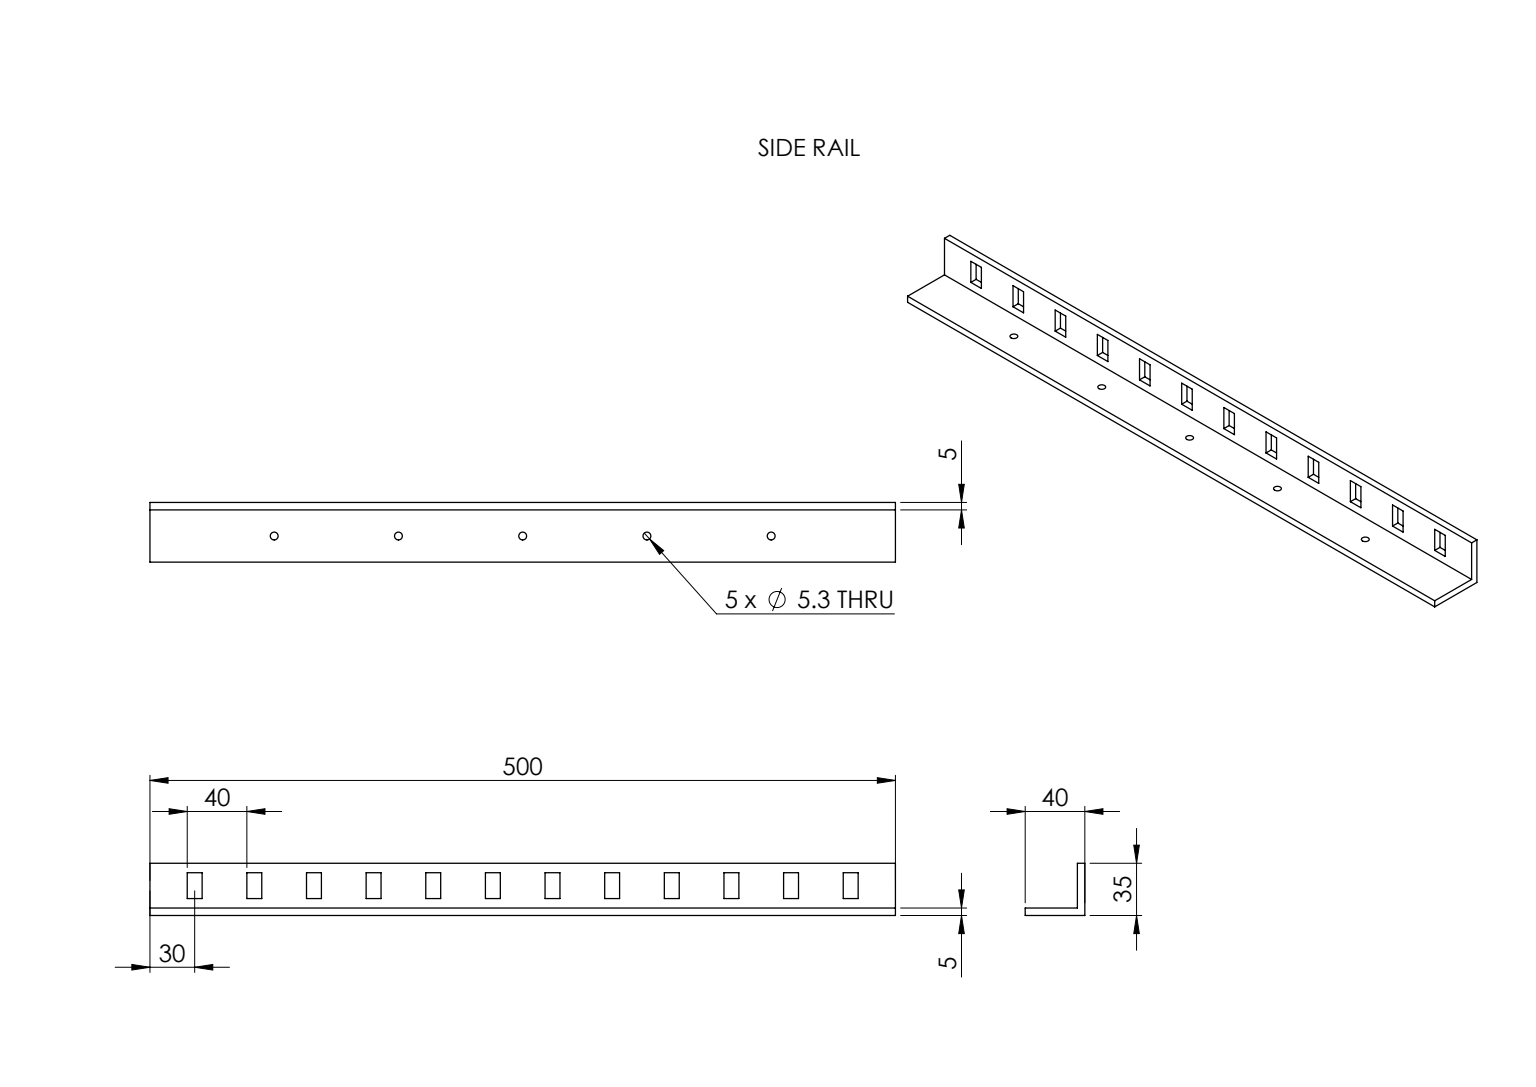
ISO-10303-21;
HEADER;
FILE_DESCRIPTION (('STEP AP214'),
    '1' );
FILE_NAME ('side rail.step',
    '2026-10-24T14:05:44',
    ( '' ),
    ( '' ),
    'SwSTEP 2.0',
    'SolidWorks 2026',
    '' );
FILE_SCHEMA (( 'AUTOMOTIVE_DESIGN' ));
ENDSEC;

DATA;
#4=CARTESIAN_POINT ( 'NONE',  ( 395.0000000000000000, -8.660254037844389075, 139.9990000000000236 ) ) ;
#6=EDGE_CURVE ( 'NONE', #1873, #4758, #4106, .T. ) ;
#9=CARTESIAN_POINT ( 'NONE',  ( 124.9999999999999858, 8.660254037844390851, 145.0000000000000284 ) ) ;
#13=EDGE_CURVE ( 'NONE', #2711, #3697, #5372, .T. ) ;
#15=DIRECTION ( 'NONE',  ( -0.000000000000000000, -0.000000000000000000, 1.000000000000000000 ) ) ;
#16=CARTESIAN_POINT ( 'NONE',  ( 395.0000000000000000, 8.660254037844390851, 140.0000000000000000 ) ) ;
#21=ORIENTED_EDGE ( 'NONE', *, *, #3815, .F. ) ;
#22=CARTESIAN_POINT ( 'NONE',  ( 445.0000000000000000, 8.660254037844390851, 145.0000000000000284 ) ) ;
#24=EDGE_CURVE ( 'NONE', #1078, #1538, #2930, .T. ) ;
#28=CARTESIAN_POINT ( 'NONE',  ( 285.0000000000000568, 8.660254037844390851, 139.9990000000000236 ) ) ;
#38=AXIS2_PLACEMENT_3D ( 'NONE', #3689, #2086, #340 ) ;
#39=DIRECTION ( 'NONE',  ( 0.000000000000000000, 0.000000000000000000, -1.000000000000000000 ) ) ;
#44=LINE ( 'NONE', #6748, #4124 ) ;
#49=CARTESIAN_POINT ( 'NONE',  ( 0.000000000000000000, -15.00000000000000000, 145.0000000000000284 ) ) ;
#50=CARTESIAN_POINT ( 'NONE',  ( 445.0000000000000000, 8.660254037844390851, 140.0000000000000000 ) ) ;
#54=EDGE_CURVE ( 'NONE', #6404, #2818, #2960, .T. ) ;
#58=VECTOR ( 'NONE', #6647, 1000.000000000000000 ) ;
#59=AXIS2_PLACEMENT_3D ( 'NONE', #3524, #1675, #1876 ) ;
#63=DIRECTION ( 'NONE',  ( 0.000000000000000000, -1.000000000000000000, 0.000000000000000000 ) ) ;
#67=EDGE_CURVE ( 'NONE', #3261, #4228, #2370, .T. ) ;
#74=LINE ( 'NONE', #2335, #4027 ) ;
#79=CARTESIAN_POINT ( 'NONE',  ( 303.3333333333333144, -20.00000000000000000, 162.5000000000000853 ) ) ;
#84=VERTEX_POINT ( 'NONE', #1298 ) ;
#90=CARTESIAN_POINT ( 'NONE',  ( 435.0000000000000568, 8.660254037844390851, 140.0000000000000000 ) ) ;
#92=ORIENTED_EDGE ( 'NONE', *, *, #7290, .F. ) ;
#95=ORIENTED_EDGE ( 'NONE', *, *, #13, .T. ) ;
#96=EDGE_CURVE ( 'NONE', #3309, #6744, #6473, .T. ) ;
#99=CARTESIAN_POINT ( 'NONE',  ( 155.0000000000000000, -8.660254037844389075, 139.9990000000000236 ) ) ;
#102=ORIENTED_EDGE ( 'NONE', *, *, #2735, .T. ) ;
#106=CARTESIAN_POINT ( 'NONE',  ( 155.0000000000000000, 8.660254037844390851, 140.0000000000000000 ) ) ;
#109=PLANE ( 'NONE',  #1833 ) ;
#110=DIRECTION ( 'NONE',  ( -0.000000000000000000, -0.000000000000000000, 1.000000000000000000 ) ) ;
#111=ORIENTED_EDGE ( 'NONE', *, *, #1690, .F. ) ;
#131=DIRECTION ( 'NONE',  ( 0.000000000000000000, -1.000000000000000000, 0.000000000000000000 ) ) ;
#133=VECTOR ( 'NONE', #4306, 1000.000000000000000 ) ;
#135=ORIENTED_EDGE ( 'NONE', *, *, #6168, .F. ) ;
#142=AXIS2_PLACEMENT_3D ( 'NONE', #4791, #2425, #751 ) ;
#152=DIRECTION ( 'NONE',  ( -0.000000000000000000, 1.000000000000000000, 0.000000000000000000 ) ) ;
#155=VECTOR ( 'NONE', #4751, 1000.000000000000000 ) ;
#157=DIRECTION ( 'NONE',  ( 0.000000000000000000, 1.000000000000000000, 0.000000000000000000 ) ) ;
#161=ORIENTED_EDGE ( 'NONE', *, *, #6818, .T. ) ;
#165=CARTESIAN_POINT ( 'NONE',  ( 84.99999999999998579, 8.660254037844390851, 145.0000000000000284 ) ) ;
#169=( GEOMETRIC_REPRESENTATION_CONTEXT ( 3 ) GLOBAL_UNCERTAINTY_ASSIGNED_CONTEXT ( ( #1828 ) ) GLOBAL_UNIT_ASSIGNED_CONTEXT ( ( #2358, #5677, #5718 ) ) REPRESENTATION_CONTEXT ( 'NONE', 'WORKASPACE' ) );
#176=VECTOR ( 'NONE', #5935, 1000.000000000000000 ) ;
#183=VERTEX_POINT ( 'NONE', #4979 ) ;
#190=VECTOR ( 'NONE', #1081, 1000.000000000000000 ) ;
#193=EDGE_CURVE ( 'NONE', #2007, #224, #1714, .T. ) ;
#194=CARTESIAN_POINT ( 'NONE',  ( 114.9999999999999858, -8.660254037844389075, 145.0000000000000284 ) ) ;
#197=CARTESIAN_POINT ( 'NONE',  ( 470.0000000000000000, 0.000000000000000000, 140.0000000000000000 ) ) ;
#201=ORIENTED_EDGE ( 'NONE', *, *, #1503, .T. ) ;
#206=LINE ( 'NONE', #6379, #2632 ) ;
#210=VECTOR ( 'NONE', #6991, 1000.000000000000000 ) ;
#211=CARTESIAN_POINT ( 'NONE',  ( 205.0000000000000284, -8.660254037844389075, 139.9990000000000236 ) ) ;
#212=LINE ( 'NONE', #4197, #176 ) ;
#218=LINE ( 'NONE', #669, #6668 ) ;
#222=DIRECTION ( 'NONE',  ( 1.000000000000000000, 0.000000000000000000, 0.000000000000000000 ) ) ;
#223=ADVANCED_FACE ( 'NONE', ( #7142 ), #1996, .F. ) ;
#224=VERTEX_POINT ( 'NONE', #6579 ) ;
#225=CARTESIAN_POINT ( 'NONE',  ( 136.6666666666666288, -15.00000000000000000, 162.5000000000000853 ) ) ;
#226=ORIENTED_EDGE ( 'NONE', *, *, #2907, .F. ) ;
#227=DIRECTION ( 'NONE',  ( 0.000000000000000000, -0.000000000000000000, 1.000000000000000000 ) ) ;
#229=CARTESIAN_POINT ( 'NONE',  ( 75.00000000000001421, -8.660254037844389075, 145.0000000000000284 ) ) ;
#234=EDGE_CURVE ( 'NONE', #6037, #2259, #3253, .T. ) ;
#236=ORIENTED_EDGE ( 'NONE', *, *, #593, .T. ) ;
#237=ORIENTED_EDGE ( 'NONE', *, *, #4529, .F. ) ;
#238=DIRECTION ( 'NONE',  ( 1.000000000000000000, 0.000000000000000000, 0.000000000000000000 ) ) ;
#239=CARTESIAN_POINT ( 'NONE',  ( 285.0000000000000568, -8.660254037844389075, 140.0000000000000000 ) ) ;
#241=CARTESIAN_POINT ( 'NONE',  ( 0.000000000000000000, 15.00000000000000000, 145.0000000000000284 ) ) ;
#244=ADVANCED_FACE ( 'NONE', ( #3311 ), #5610, .F. ) ;
#245=EDGE_LOOP ( 'NONE', ( #1865, #2331, #5916, #510 ) ) ;
#246=LINE ( 'NONE', #1986, #5667 ) ;
#247=EDGE_LOOP ( 'NONE', ( #1984, #1651 ) ) ;
#250=DIRECTION ( 'NONE',  ( -0.000000000000000000, -0.000000000000000000, 1.000000000000000000 ) ) ;
#254=AXIS2_PLACEMENT_3D ( 'NONE', #4363, #7167, #6172 ) ;
#257=CARTESIAN_POINT ( 'NONE',  ( 315.0000000000000568, -8.660254037844389075, 140.0000000000000000 ) ) ;
#258=DIRECTION ( 'NONE',  ( 0.000000000000000000, 0.000000000000000000, 1.000000000000000000 ) ) ;
#261=CARTESIAN_POINT ( 'NONE',  ( 155.0000000000000000, -8.660254037844389075, 140.0000000000000000 ) ) ;
#263=FACE_OUTER_BOUND ( 'NONE', #980, .T. ) ;
#264=FACE_BOUND ( 'NONE', #5011, .T. ) ;
#266=VERTEX_POINT ( 'NONE', #5591 ) ;
#268=VECTOR ( 'NONE', #2901, 1000.000000000000000 ) ;
#270=EDGE_LOOP ( 'NONE', ( #4562, #2642, #3937, #2477 ) ) ;
#272=CARTESIAN_POINT ( 'NONE',  ( -30.00000000000000000, 0.000000000000000000, 145.0000000000000284 ) ) ;
#274=LINE ( 'NONE', #4831, #5071 ) ;
#275=LINE ( 'NONE', #241, #3751 ) ;
#276=ADVANCED_FACE ( 'NONE', ( #508 ), #4512, .F. ) ;
#289=FACE_OUTER_BOUND ( 'NONE', #1974, .T. ) ;
#291=VECTOR ( 'NONE', #1291, 1000.000000000000000 ) ;
#295=DIRECTION ( 'NONE',  ( 0.000000000000000000, 1.000000000000000000, 0.000000000000000000 ) ) ;
#304=CARTESIAN_POINT ( 'NONE',  ( 35.00000000000000000, -8.660254037844389075, 145.0000000000000284 ) ) ;
#305=VECTOR ( 'NONE', #531, 1000.000000000000000 ) ;
#307=EDGE_LOOP ( 'NONE', ( #1128, #3991, #4538, #5321 ) ) ;
#309=ORIENTED_EDGE ( 'NONE', *, *, #948, .F. ) ;
#310=VERTEX_POINT ( 'NONE', #3745 ) ;
#314=AXIS2_PLACEMENT_3D ( 'NONE', #1589, #3208, #5511 ) ;
#315=LINE ( 'NONE', #4230, #906 ) ;
#319=EDGE_CURVE ( 'NONE', #5864, #3377, #5467, .T. ) ;
#322=ORIENTED_EDGE ( 'NONE', *, *, #1493, .T. ) ;
#323=PLANE ( 'NONE',  #7068 ) ;
#325=ORIENTED_EDGE ( 'NONE', *, *, #3553, .T. ) ;
#327=DIRECTION ( 'NONE',  ( 0.000000000000000000, -0.000000000000000000, 1.000000000000000000 ) ) ;
#330=ORIENTED_EDGE ( 'NONE', *, *, #694, .F. ) ;
#335=CARTESIAN_POINT ( 'NONE',  ( 35.00000000000000000, 8.660254037844390851, 140.0000000000000000 ) ) ;
#340=DIRECTION ( 'NONE',  ( 0.000000000000000000, -0.000000000000000000, -1.000000000000000000 ) ) ;
#341=DIRECTION ( 'NONE',  ( -1.000000000000000000, 0.000000000000000000, 0.000000000000000000 ) ) ;
#343=ORIENTED_EDGE ( 'NONE', *, *, #1444, .F. ) ;
#347=EDGE_LOOP ( 'NONE', ( #5848, #2567, #5256, #892 ) ) ;
#357=ORIENTED_EDGE ( 'NONE', *, *, #1783, .F. ) ;
#367=CARTESIAN_POINT ( 'NONE',  ( 355.0000000000000000, -8.660254037844389075, 145.0000000000000284 ) ) ;
#368=EDGE_CURVE ( 'NONE', #3826, #310, #7198, .T. ) ;
#372=EDGE_LOOP ( 'NONE', ( #4500, #2241, #5481, #4153 ) ) ;
#373=VECTOR ( 'NONE', #1246, 1000.000000000000000 ) ;
#376=DIRECTION ( 'NONE',  ( 1.000000000000000000, 0.000000000000000000, 0.000000000000000000 ) ) ;
#377=FACE_BOUND ( 'NONE', #5167, .T. ) ;
#382=AXIS2_PLACEMENT_3D ( 'NONE', #5714, #6317, #1103 ) ;
#383=EDGE_LOOP ( 'NONE', ( #6223, #1224 ) ) ;
#388=CARTESIAN_POINT ( 'NONE',  ( 315.0000000000000568, -8.660254037844389075, 145.0000000000000284 ) ) ;
#398=LINE ( 'NONE', #994, #4132 ) ;
#401=LINE ( 'NONE', #3139, #1706 ) ;
#406=EDGE_LOOP ( 'NONE', ( #4251, #4299, #5740, #309 ) ) ;
#409=CARTESIAN_POINT ( 'NONE',  ( 4.999999999999999112, -8.660254037844389075, 140.0000000000000000 ) ) ;
#419=EDGE_CURVE ( 'NONE', #6751, #183, #6215, .T. ) ;
#427=VECTOR ( 'NONE', #131, 1000.000000000000000 ) ;
#433=DIRECTION ( 'NONE',  ( -0.000000000000000000, 1.000000000000000000, -0.000000000000000000 ) ) ;
#434=DIRECTION ( 'NONE',  ( -1.000000000000000000, 0.000000000000000000, -0.000000000000000000 ) ) ;
#441=ORIENTED_EDGE ( 'NONE', *, *, #1230, .T. ) ;
#443=FACE_OUTER_BOUND ( 'NONE', #2972, .T. ) ;
#444=CARTESIAN_POINT ( 'NONE',  ( 164.9999999999999716, 8.660254037844390851, 145.0000000000000284 ) ) ;
#446=CARTESIAN_POINT ( 'NONE',  ( 285.0000000000000568, 8.660254037844390851, 140.0000000000000000 ) ) ;
#453=CIRCLE ( 'NONE', #2820, 2.649999999999985700 ) ;
#458=ORIENTED_EDGE ( 'NONE', *, *, #67, .F. ) ;
#464=DIRECTION ( 'NONE',  ( -0.000000000000000000, 1.000000000000000000, -0.000000000000000000 ) ) ;
#466=ORIENTED_EDGE ( 'NONE', *, *, #7136, .F. ) ;
#467=LINE ( 'NONE', #1023, #7209 ) ;
#469=ORIENTED_EDGE ( 'NONE', *, *, #956, .F. ) ;
#472=PLANE ( 'NONE',  #1920 ) ;
#474=EDGE_CURVE ( 'NONE', #2018, #3309, #212, .T. ) ;
#479=FACE_BOUND ( 'NONE', #3779, .T. ) ;
#485=FACE_OUTER_BOUND ( 'NONE', #5786, .T. ) ;
#491=CARTESIAN_POINT ( 'NONE',  ( 435.0000000000000568, -8.660254037844389075, 145.0000000000000284 ) ) ;
#492=LINE ( 'NONE', #3348, #3419 ) ;
#494=DIRECTION ( 'NONE',  ( -0.000000000000000000, -0.000000000000000000, 1.000000000000000000 ) ) ;
#505=CARTESIAN_POINT ( 'NONE',  ( 275.0000000000000000, 8.660254037844390851, 140.0000000000000000 ) ) ;
#508=FACE_OUTER_BOUND ( 'NONE', #5725, .T. ) ;
#509=LINE ( 'NONE', #3410, #7223 ) ;
#510=ORIENTED_EDGE ( 'NONE', *, *, #4260, .T. ) ;
#514=LINE ( 'NONE', #2355, #1215 ) ;
#515=FACE_BOUND ( 'NONE', #4736, .T. ) ;
#516=DIRECTION ( 'NONE',  ( -0.000000000000000000, -0.000000000000000000, 1.000000000000000000 ) ) ;
#519=EDGE_LOOP ( 'NONE', ( #3409, #1674, #1856, #6245 ) ) ;
#524=PLANE ( 'NONE',  #3519 ) ;
#525=AXIS2_PLACEMENT_3D ( 'NONE', #3543, #4080, #2381 ) ;
#527=ORIENTED_EDGE ( 'NONE', *, *, #701, .F. ) ;
#528=CARTESIAN_POINT ( 'NONE',  ( 155.0000000000000000, 8.660254037844390851, 139.9990000000000236 ) ) ;
#529=CARTESIAN_POINT ( 'NONE',  ( 235.0000000000000000, 8.660254037844390851, 140.0000000000000000 ) ) ;
#531=DIRECTION ( 'NONE',  ( 0.000000000000000000, -1.000000000000000000, 0.000000000000000000 ) ) ;
#532=VECTOR ( 'NONE', #4257, 1000.000000000000000 ) ;
#535=DIRECTION ( 'NONE',  ( 0.000000000000000000, 1.000000000000000000, 0.000000000000000000 ) ) ;
#538=LINE ( 'NONE', #6204, #2789 ) ;
#539=AXIS2_PLACEMENT_3D ( 'NONE', #7178, #4930, #2078 ) ;
#542=LINE ( 'NONE', #49, #3343 ) ;
#547=STYLED_ITEM ( 'NONE', ( #4320 ), #5754 ) ;
#550=ORIENTED_EDGE ( 'NONE', *, *, #6741, .T. ) ;
#551=VECTOR ( 'NONE', #6256, 1000.000000000000000 ) ;
#553=FACE_OUTER_BOUND ( 'NONE', #3654, .T. ) ;
#554=CARTESIAN_POINT ( 'NONE',  ( 303.3333333333333144, -14.99999999999999822, 162.5000000000000853 ) ) ;
#556=EDGE_CURVE ( 'NONE', #1367, #3466, #7089, .T. ) ;
#559=VECTOR ( 'NONE', #1074, 1000.000000000000000 ) ;
#561=EDGE_LOOP ( 'NONE', ( #5979, #4892 ) ) ;
#564=VECTOR ( 'NONE', #6045, 1000.000000000000000 ) ;
#573=VECTOR ( 'NONE', #3455, 1000.000000000000000 ) ;
#576=ORIENTED_EDGE ( 'NONE', *, *, #6862, .T. ) ;
#583=DIRECTION ( 'NONE',  ( 0.000000000000000000, 0.000000000000000000, -1.000000000000000000 ) ) ;
#584=VERTEX_POINT ( 'NONE', #1395 ) ;
#588=CARTESIAN_POINT ( 'NONE',  ( 386.6666666666666288, -14.99999999999999822, 162.5000000000000853 ) ) ;
#591=ORIENTED_EDGE ( 'NONE', *, *, #1590, .T. ) ;
#593=EDGE_CURVE ( 'NONE', #7027, #310, #2577, .T. ) ;
#595=ORIENTED_EDGE ( 'NONE', *, *, #5293, .F. ) ;
#596=LINE ( 'NONE', #3885, #190 ) ;
#601=CARTESIAN_POINT ( 'NONE',  ( 470.0000000000000000, -15.00000000000000000, 145.0000000000000284 ) ) ;
#604=EDGE_LOOP ( 'NONE', ( #960, #1830, #4158, #6314 ) ) ;
#606=ORIENTED_EDGE ( 'NONE', *, *, #2840, .T. ) ;
#607=AXIS2_PLACEMENT_3D ( 'NONE', #5873, #2374, #227 ) ;
#612=ORIENTED_EDGE ( 'NONE', *, *, #6327, .F. ) ;
#615=EDGE_LOOP ( 'NONE', ( #7175, #5759 ) ) ;
#617=DIRECTION ( 'NONE',  ( -1.000000000000000000, 0.000000000000000000, 0.000000000000000000 ) ) ;
#618=PLANE ( 'NONE',  #6780 ) ;
#628=DIRECTION ( 'NONE',  ( 0.000000000000000000, 0.000000000000000000, 1.000000000000000000 ) ) ;
#635=EDGE_CURVE ( 'NONE', #3059, #1111, #1755, .T. ) ;
#636=ORIENTED_EDGE ( 'NONE', *, *, #5776, .F. ) ;
#642=VECTOR ( 'NONE', #4176, 1000.000000000000000 ) ;
#643=DIRECTION ( 'NONE',  ( 0.000000000000000000, 0.000000000000000000, -1.000000000000000000 ) ) ;
#644=LINE ( 'NONE', #2899, #2333 ) ;
#645=CARTESIAN_POINT ( 'NONE',  ( 235.0000000000000000, 8.660254037844390851, 139.9990000000000236 ) ) ;
#646=FACE_OUTER_BOUND ( 'NONE', #5518, .T. ) ;
#648=EDGE_CURVE ( 'NONE', #4019, #2725, #2787, .T. ) ;
#651=VECTOR ( 'NONE', #2504, 1000.000000000000000 ) ;
#652=EDGE_CURVE ( 'NONE', #2249, #3158, #5654, .T. ) ;
#662=COLOUR_RGB ( '',0.8941176470588234615, 0.8941176470588234615, 0.8941176470588234615 ) ;
#664=ORIENTED_EDGE ( 'NONE', *, *, #319, .T. ) ;
#666=LINE ( 'NONE', #6392, #5923 ) ;
#668=VECTOR ( 'NONE', #3036, 1000.000000000000000 ) ;
#669=CARTESIAN_POINT ( 'NONE',  ( 435.0000000000000568, 8.660254037844390851, 139.9990000000000236 ) ) ;
#675=CIRCLE ( 'NONE', #5109, 2.649999999999985700 ) ;
#677=LINE ( 'NONE', #3608, #2568 ) ;
#683=CARTESIAN_POINT ( 'NONE',  ( 219.9999999999999716, -15.00000000000000000, 159.8500000000001080 ) ) ;
#684=PLANE ( 'NONE',  #1220 ) ;
#685=CARTESIAN_POINT ( 'NONE',  ( 205.0000000000000284, -8.660254037844389075, 140.0000000000000000 ) ) ;
#687=ORIENTED_EDGE ( 'NONE', *, *, #4021, .F. ) ;
#690=CARTESIAN_POINT ( 'NONE',  ( 275.0000000000000000, 8.660254037844390851, 139.9990000000000236 ) ) ;
#694=EDGE_CURVE ( 'NONE', #7258, #2062, #2271, .T. ) ;
#696=ORIENTED_EDGE ( 'NONE', *, *, #5063, .T. ) ;
#697=EDGE_LOOP ( 'NONE', ( #5882, #6378, #4879, #7072 ) ) ;
#701=EDGE_CURVE ( 'NONE', #2491, #3982, #2202, .T. ) ;
#702=LINE ( 'NONE', #1658, #4364 ) ;
#703=CARTESIAN_POINT ( 'NONE',  ( 470.0000000000000000, 15.00000000000000000, 145.0000000000000284 ) ) ;
#704=ORIENTED_EDGE ( 'NONE', *, *, #4059, .T. ) ;
#708=DIRECTION ( 'NONE',  ( 0.000000000000000000, -1.000000000000000000, 0.000000000000000000 ) ) ;
#713=DIRECTION ( 'NONE',  ( -1.000000000000000000, 0.000000000000000000, -0.000000000000000000 ) ) ;
#715=EDGE_LOOP ( 'NONE', ( #2151, #1356, #4570, #1862 ) ) ;
#717=EDGE_CURVE ( 'NONE', #5864, #5089, #2077, .T. ) ;
#726=DIRECTION ( 'NONE',  ( 0.000000000000000000, 0.000000000000000000, 1.000000000000000000 ) ) ;
#728=EDGE_CURVE ( 'NONE', #7155, #3466, #4536, .T. ) ;
#729=ORIENTED_EDGE ( 'NONE', *, *, #2396, .T. ) ;
#730=VECTOR ( 'NONE', #6726, 1000.000000000000000 ) ;
#731=DIRECTION ( 'NONE',  ( -0.000000000000000000, 0.000000000000000000, 1.000000000000000000 ) ) ;
#732=VERTEX_POINT ( 'NONE', #3972 ) ;
#733=AXIS2_PLACEMENT_3D ( 'NONE', #3013, #238, #4760 ) ;
#736=ORIENTED_EDGE ( 'NONE', *, *, #635, .F. ) ;
#737=LINE ( 'NONE', #1881, #668 ) ;
#738=VECTOR ( 'NONE', #3505, 1000.000000000000000 ) ;
#741=ORIENTED_EDGE ( 'NONE', *, *, #4255, .F. ) ;
#742=VECTOR ( 'NONE', #3862, 1000.000000000000000 ) ;
#743=LINE ( 'NONE', #3044, #5257 ) ;
#747=ORIENTED_EDGE ( 'NONE', *, *, #1925, .T. ) ;
#751=DIRECTION ( 'NONE',  ( 0.000000000000000000, -0.000000000000000000, -1.000000000000000000 ) ) ;
#767=VERTEX_POINT ( 'NONE', #2448 ) ;
#771=DIRECTION ( 'NONE',  ( -0.000000000000000000, -0.000000000000000000, 1.000000000000000000 ) ) ;
#772=UNCERTAINTY_MEASURE_WITH_UNIT (LENGTH_MEASURE( 1.000000000000000082E-05 ), #4843, 'distance_accuracy_value', 'NONE');
#776=VECTOR ( 'NONE', #5437, 1000.000000000000000 ) ;
#777=CARTESIAN_POINT ( 'NONE',  ( 355.0000000000000000, 8.660254037844390851, 140.0000000000000000 ) ) ;
#779=ORIENTED_EDGE ( 'NONE', *, *, #4287, .T. ) ;
#782=AXIS2_PLACEMENT_3D ( 'NONE', #1402, #5977, #5942 ) ;
#788=ADVANCED_FACE ( 'NONE', ( #5803 ), #2341, .F. ) ;
#806=CARTESIAN_POINT ( 'NONE',  ( 35.00000000000000000, 8.660254037844390851, 145.0000000000000284 ) ) ;
#809=EDGE_CURVE ( 'NONE', #1731, #4768, #4779, .T. ) ;
#811=EDGE_LOOP ( 'NONE', ( #6572, #6291, #4914, #5894 ) ) ;
#812=LINE ( 'NONE', #2511, #1454 ) ;
#814=LINE ( 'NONE', #4326, #5802 ) ;
#816=ORIENTED_EDGE ( 'NONE', *, *, #3949, .T. ) ;
#818=VERTEX_POINT ( 'NONE', #2961 ) ;
#819=EDGE_CURVE ( 'NONE', #4268, #3509, #677, .T. ) ;
#825=CARTESIAN_POINT ( 'NONE',  ( 75.00000000000001421, -8.660254037844389075, 140.0000000000000000 ) ) ;
#826=ADVANCED_FACE ( 'NONE', ( #5951 ), #5268, .F. ) ;
#828=VERTEX_POINT ( 'NONE', #1883 ) ;
#839=DIRECTION ( 'NONE',  ( 0.000000000000000000, -0.000000000000000000, 1.000000000000000000 ) ) ;
#846=FACE_OUTER_BOUND ( 'NONE', #2317, .T. ) ;
#863=CARTESIAN_POINT ( 'NONE',  ( -30.00000000000002842, -20.00000000000000000, 140.0000000000000000 ) ) ;
#873=DIRECTION ( 'NONE',  ( -0.000000000000000000, -0.000000000000000000, 1.000000000000000000 ) ) ;
#875=ORIENTED_EDGE ( 'NONE', *, *, #1964, .T. ) ;
#884=ORIENTED_EDGE ( 'NONE', *, *, #6060, .F. ) ;
#886=ORIENTED_EDGE ( 'NONE', *, *, #956, .T. ) ;
#888=PLANE ( 'NONE',  #6650 ) ;
#892=ORIENTED_EDGE ( 'NONE', *, *, #728, .F. ) ;
#897=LINE ( 'NONE', #936, #3507 ) ;
#898=AXIS2_PLACEMENT_3D ( 'NONE', #964, #929, #5484 ) ;
#900=ORIENTED_EDGE ( 'NONE', *, *, #6139, .F. ) ;
#903=EDGE_LOOP ( 'NONE', ( #1637, #4277, #2481, #4578 ) ) ;
#905=CARTESIAN_POINT ( 'NONE',  ( 53.33333333333330017, -14.99999999999999822, 159.8500000000001080 ) ) ;
#906=VECTOR ( 'NONE', #6488, 1000.000000000000000 ) ;
#909=LINE ( 'NONE', #5430, #6286 ) ;
#910=CARTESIAN_POINT ( 'NONE',  ( 53.33333333333330017, -15.00000000000000000, 165.1500000000000625 ) ) ;
#913=VECTOR ( 'NONE', #5806, 1000.000000000000000 ) ;
#914=ORIENTED_EDGE ( 'NONE', *, *, #920, .T. ) ;
#915=ADVANCED_FACE ( 'NONE', ( #846 ), #6580, .F. ) ;
#920=EDGE_CURVE ( 'NONE', #1078, #2826, #2516, .T. ) ;
#924=LINE ( 'NONE', #7256, #3423 ) ;
#925=ORIENTED_EDGE ( 'NONE', *, *, #2603, .F. ) ;
#928=ORIENTED_EDGE ( 'NONE', *, *, #2272, .F. ) ;
#929=DIRECTION ( 'NONE',  ( 0.000000000000000000, 1.000000000000000000, 0.000000000000000000 ) ) ;
#932=VERTEX_POINT ( 'NONE', #6625 ) ;
#934=FACE_OUTER_BOUND ( 'NONE', #4798, .T. ) ;
#936=CARTESIAN_POINT ( 'NONE',  ( 325.0000000000000000, 8.660254037844390851, 145.0000000000000284 ) ) ;
#945=CARTESIAN_POINT ( 'NONE',  ( -5.000000000000000888, -8.660254037844389075, 145.0000000000000284 ) ) ;
#947=CARTESIAN_POINT ( 'NONE',  ( 365.0000000000000000, 8.660254037844390851, 139.9990000000000236 ) ) ;
#948=EDGE_CURVE ( 'NONE', #4387, #2711, #5451, .T. ) ;
#952=ORIENTED_EDGE ( 'NONE', *, *, #1964, .F. ) ;
#953=CARTESIAN_POINT ( 'NONE',  ( 195.0000000000000000, 8.660254037844390851, 145.0000000000000284 ) ) ;
#954=DIRECTION ( 'NONE',  ( 0.000000000000000000, -1.000000000000000000, 0.000000000000000000 ) ) ;
#955=DIRECTION ( 'NONE',  ( -0.000000000000000000, 1.000000000000000000, -0.000000000000000000 ) ) ;
#956=EDGE_CURVE ( 'NONE', #6406, #3386, #3684, .T. ) ;
#960=ORIENTED_EDGE ( 'NONE', *, *, #4756, .F. ) ;
#963=EDGE_LOOP ( 'NONE', ( #3170, #5909, #4292, #1829 ) ) ;
#964=CARTESIAN_POINT ( 'NONE',  ( 136.6666666666666288, -20.00000000000000000, 162.5000000000000853 ) ) ;
#969=ORIENTED_EDGE ( 'NONE', *, *, #234, .T. ) ;
#974=FACE_BOUND ( 'NONE', #903, .T. ) ;
#980=EDGE_LOOP ( 'NONE', ( #1441, #2729, #2992, #5121 ) ) ;
#985=LINE ( 'NONE', #2099, #3236 ) ;
#986=DIRECTION ( 'NONE',  ( -1.000000000000000000, -0.000000000000000000, -0.000000000000000000 ) ) ;
#990=LINE ( 'NONE', #3293, #3256 ) ;
#994=CARTESIAN_POINT ( 'NONE',  ( 114.9999999999999858, 8.660254037844390851, 140.0000000000000000 ) ) ;
#999=DIRECTION ( 'NONE',  ( -0.000000000000000000, -0.000000000000000000, 1.000000000000000000 ) ) ;
#1001=ORIENTED_EDGE ( 'NONE', *, *, #3815, .T. ) ;
#1011=ORIENTED_EDGE ( 'NONE', *, *, #5466, .T. ) ;
#1014=EDGE_CURVE ( 'NONE', #5089, #5864, #453, .T. ) ;
#1023=CARTESIAN_POINT ( 'NONE',  ( 45.00000000000000000, 8.660254037844390851, 139.9990000000000236 ) ) ;
#1024=ORIENTED_EDGE ( 'NONE', *, *, #3658, .F. ) ;
#1025=ORIENTED_EDGE ( 'NONE', *, *, #5063, .F. ) ;
#1030=LINE ( 'NONE', #3289, #2044 ) ;
#1033=FACE_OUTER_BOUND ( 'NONE', #3956, .T. ) ;
#1034=VECTOR ( 'NONE', #5723, 1000.000000000000000 ) ;
#1035=ORIENTED_EDGE ( 'NONE', *, *, #7145, .F. ) ;
#1036=CIRCLE ( 'NONE', #1847, 2.649999999999985700 ) ;
#1039=LINE ( 'NONE', #2109, #7181 ) ;
#1041=VECTOR ( 'NONE', #157, 1000.000000000000000 ) ;
#1049=EDGE_CURVE ( 'NONE', #6322, #1596, #6310, .T. ) ;
#1052=ORIENTED_EDGE ( 'NONE', *, *, #819, .T. ) ;
#1056=DIRECTION ( 'NONE',  ( -0.000000000000000000, 1.000000000000000000, -0.000000000000000000 ) ) ;
#1061=ORIENTED_EDGE ( 'NONE', *, *, #5857, .T. ) ;
#1072=DIRECTION ( 'NONE',  ( -0.000000000000000000, -0.000000000000000000, 1.000000000000000000 ) ) ;
#1074=DIRECTION ( 'NONE',  ( 0.000000000000000000, -1.000000000000000000, 0.000000000000000000 ) ) ;
#1075=CARTESIAN_POINT ( 'NONE',  ( 35.00000000000000000, -8.660254037844389075, 139.9990000000000236 ) ) ;
#1076=CYLINDRICAL_SURFACE ( 'NONE', #4002, 2.649999999999985700 ) ;
#1077=ORIENTED_EDGE ( 'NONE', *, *, #2199, .F. ) ;
#1078=VERTEX_POINT ( 'NONE', #3427 ) ;
#1081=DIRECTION ( 'NONE',  ( 0.000000000000000000, -1.000000000000000000, 0.000000000000000000 ) ) ;
#1084=VERTEX_POINT ( 'NONE', #3312 ) ;
#1087=LINE ( 'NONE', #2161, #5433 ) ;
#1095=ORIENTED_EDGE ( 'NONE', *, *, #6194, .T. ) ;
#1101=FACE_OUTER_BOUND ( 'NONE', #7030, .T. ) ;
#1103=DIRECTION ( 'NONE',  ( 0.000000000000000000, -0.000000000000000000, -1.000000000000000000 ) ) ;
#1107=ADVANCED_FACE ( 'NONE', ( #5095 ), #3964, .F. ) ;
#1110=ORIENTED_EDGE ( 'NONE', *, *, #1503, .F. ) ;
#1111=VERTEX_POINT ( 'NONE', #3887 ) ;
#1114=ORIENTED_EDGE ( 'NONE', *, *, #6818, .F. ) ;
#1115=EDGE_CURVE ( 'NONE', #3386, #84, #6853, .T. ) ;
#1118=CARTESIAN_POINT ( 'NONE',  ( 470.0000000000000000, -15.00000000000000000, 180.0000000000000284 ) ) ;
#1128=ORIENTED_EDGE ( 'NONE', *, *, #1710, .T. ) ;
#1138=VECTOR ( 'NONE', #1649, 1000.000000000000000 ) ;
#1139=ORIENTED_EDGE ( 'NONE', *, *, #3973, .T. ) ;
#1152=ORIENTED_EDGE ( 'NONE', *, *, #3553, .F. ) ;
#1153=EDGE_CURVE ( 'NONE', #932, #266, #492, .T. ) ;
#1157=DIRECTION ( 'NONE',  ( -1.000000000000000000, 0.000000000000000000, -0.000000000000000000 ) ) ;
#1158=DIRECTION ( 'NONE',  ( -0.000000000000000000, 1.000000000000000000, -0.000000000000000000 ) ) ;
#1159=EDGE_CURVE ( 'NONE', #1397, #2205, #2191, .T. ) ;
#1165=DIRECTION ( 'NONE',  ( -0.000000000000000000, -0.000000000000000000, 1.000000000000000000 ) ) ;
#1166=VECTOR ( 'NONE', #250, 1000.000000000000000 ) ;
#1168=VERTEX_POINT ( 'NONE', #1118 ) ;
#1175=CARTESIAN_POINT ( 'NONE',  ( 164.9999999999999716, 8.660254037844390851, 139.9990000000000236 ) ) ;
#1181=DIRECTION ( 'NONE',  ( 0.000000000000000000, 1.000000000000000000, 0.000000000000000000 ) ) ;
#1191=ADVANCED_FACE ( 'NONE', ( #1775 ), #5192, .F. ) ;
#1192=CARTESIAN_POINT ( 'NONE',  ( 35.00000000000000000, -8.660254037844389075, 139.9990000000000236 ) ) ;
#1196=CARTESIAN_POINT ( 'NONE',  ( -30.00000000000002842, 15.00000000000000000, 145.0000000000000284 ) ) ;
#1201=ORIENTED_EDGE ( 'NONE', *, *, #4112, .F. ) ;
#1203=DIRECTION ( 'NONE',  ( -0.000000000000000000, -0.000000000000000000, 1.000000000000000000 ) ) ;
#1205=CARTESIAN_POINT ( 'NONE',  ( 395.0000000000000000, 8.660254037844390851, 145.0000000000000284 ) ) ;
#1207=VERTEX_POINT ( 'NONE', #703 ) ;
#1211=CARTESIAN_POINT ( 'NONE',  ( 386.6666666666666288, -20.00000000000000000, 162.5000000000000853 ) ) ;
#1212=VECTOR ( 'NONE', #3174, 1000.000000000000000 ) ;
#1213=CARTESIAN_POINT ( 'NONE',  ( 315.0000000000000568, 8.660254037844390851, 140.0000000000000000 ) ) ;
#1214=FACE_BOUND ( 'NONE', #347, .T. ) ;
#1215=VECTOR ( 'NONE', #6879, 1000.000000000000000 ) ;
#1216=CARTESIAN_POINT ( 'NONE',  ( 235.0000000000000000, -8.660254037844389075, 145.0000000000000284 ) ) ;
#1217=ORIENTED_EDGE ( 'NONE', *, *, #7290, .T. ) ;
#1220=AXIS2_PLACEMENT_3D ( 'NONE', #4115, #2935, #3077 ) ;
#1221=LINE ( 'NONE', #5794, #210 ) ;
#1222=EDGE_CURVE ( 'NONE', #3817, #5003, #74, .T. ) ;
#1223=VECTOR ( 'NONE', #494, 1000.000000000000000 ) ;
#1224=ORIENTED_EDGE ( 'NONE', *, *, #4343, .T. ) ;
#1227=ORIENTED_EDGE ( 'NONE', *, *, #3658, .T. ) ;
#1229=ORIENTED_EDGE ( 'NONE', *, *, #5799, .T. ) ;
#1230=EDGE_CURVE ( 'NONE', #6875, #584, #3489, .T. ) ;
#1237=EDGE_LOOP ( 'NONE', ( #4346, #2604, #5037, #3051 ) ) ;
#1240=EDGE_CURVE ( 'NONE', #2491, #4387, #1221, .T. ) ;
#1244=AXIS2_PLACEMENT_3D ( 'NONE', #947, #3203, #2653 ) ;
#1246=DIRECTION ( 'NONE',  ( -1.000000000000000000, -0.000000000000000000, -0.000000000000000000 ) ) ;
#1248=EDGE_CURVE ( 'NONE', #6406, #1422, #218, .T. ) ;
#1251=VECTOR ( 'NONE', #1924, 1000.000000000000000 ) ;
#1256=DIRECTION ( 'NONE',  ( -1.000000000000000000, 0.000000000000000000, -0.000000000000000000 ) ) ;
#1257=ORIENTED_EDGE ( 'NONE', *, *, #6327, .T. ) ;
#1260=VECTOR ( 'NONE', #6294, 1000.000000000000000 ) ;
#1262=AXIS2_PLACEMENT_3D ( 'NONE', #2572, #4868, #5324 ) ;
#1264=DIRECTION ( 'NONE',  ( 1.000000000000000000, 0.000000000000000000, 0.000000000000000000 ) ) ;
#1265=CARTESIAN_POINT ( 'NONE',  ( 35.00000000000000000, 8.660254037844390851, 139.9990000000000236 ) ) ;
#1267=DIRECTION ( 'NONE',  ( -0.000000000000000000, 1.000000000000000000, -0.000000000000000000 ) ) ;
#1268=ORIENTED_EDGE ( 'NONE', *, *, #1872, .F. ) ;
#1274=DIRECTION ( 'NONE',  ( -0.000000000000000000, -0.000000000000000000, 1.000000000000000000 ) ) ;
#1287=ADVANCED_FACE ( 'NONE', ( #6614 ), #7208, .F. ) ;
#1291=DIRECTION ( 'NONE',  ( 0.000000000000000000, -1.000000000000000000, 0.000000000000000000 ) ) ;
#1292=ORIENTED_EDGE ( 'NONE', *, *, #6513, .T. ) ;
#1293=EDGE_CURVE ( 'NONE', #3386, #7293, #5516, .T. ) ;
#1297=FACE_OUTER_BOUND ( 'NONE', #7119, .T. ) ;
#1298=CARTESIAN_POINT ( 'NONE',  ( 445.0000000000000000, -8.660254037844389075, 140.0000000000000000 ) ) ;
#1305=DIRECTION ( 'NONE',  ( -0.000000000000000000, 1.000000000000000000, -0.000000000000000000 ) ) ;
#1306=EDGE_CURVE ( 'NONE', #5483, #6671, #924, .T. ) ;
#1307=ORIENTED_EDGE ( 'NONE', *, *, #5165, .T. ) ;
#1308=VERTEX_POINT ( 'NONE', #5402 ) ;
#1314=DIRECTION ( 'NONE',  ( 0.000000000000000000, -0.000000000000000000, -1.000000000000000000 ) ) ;
#1319=CARTESIAN_POINT ( 'NONE',  ( 303.3333333333333144, -20.00000000000000000, 165.1500000000000625 ) ) ;
#1323=VECTOR ( 'NONE', #4650, 1000.000000000000000 ) ;
#1325=VERTEX_POINT ( 'NONE', #6660 ) ;
#1328=DIRECTION ( 'NONE',  ( 1.000000000000000000, 0.000000000000000000, 0.000000000000000000 ) ) ;
#1330=CARTESIAN_POINT ( 'NONE',  ( -30.00000000000002842, -20.00000000000000000, 180.0000000000000284 ) ) ;
#1332=ORIENTED_EDGE ( 'NONE', *, *, #4834, .F. ) ;
#1334=PLANE ( 'NONE',  #607 ) ;
#1341=LINE ( 'NONE', #3622, #6881 ) ;
#1343=AXIS2_PLACEMENT_3D ( 'NONE', #3176, #6612, #5478 ) ;
#1346=LINE ( 'NONE', #5282, #4563 ) ;
#1353=AXIS2_PLACEMENT_3D ( 'NONE', #4354, #3867, #2656 ) ;
#1354=LINE ( 'NONE', #211, #5662 ) ;
#1356=ORIENTED_EDGE ( 'NONE', *, *, #5165, .F. ) ;
#1361=CARTESIAN_POINT ( 'NONE',  ( 164.9999999999999716, -8.660254037844389075, 139.9990000000000236 ) ) ;
#1365=FACE_OUTER_BOUND ( 'NONE', #5125, .T. ) ;
#1367=VERTEX_POINT ( 'NONE', #4922 ) ;
#1368=VECTOR ( 'NONE', #5012, 1000.000000000000000 ) ;
#1373=EDGE_CURVE ( 'NONE', #7234, #3206, #3142, .T. ) ;
#1374=ORIENTED_EDGE ( 'NONE', *, *, #5945, .T. ) ;
#1375=AXIS2_PLACEMENT_3D ( 'NONE', #3460, #1328, #3565 ) ;
#1378=EDGE_LOOP ( 'NONE', ( #1421, #1139, #4693, #6522 ) ) ;
#1391=CARTESIAN_POINT ( 'NONE',  ( 275.0000000000000000, -8.660254037844389075, 140.0000000000000000 ) ) ;
#1394=FACE_OUTER_BOUND ( 'NONE', #6543, .T. ) ;
#1395=CARTESIAN_POINT ( 'NONE',  ( 84.99999999999998579, -8.660254037844389075, 145.0000000000000284 ) ) ;
#1396=AXIS2_PLACEMENT_3D ( 'NONE', #79, #2338, #4636 ) ;
#1397=VERTEX_POINT ( 'NONE', #2587 ) ;
#1402=CARTESIAN_POINT ( 'NONE',  ( 0.000000000000000000, -15.00000000000000000, 0.000000000000000000 ) ) ;
#1403=EDGE_LOOP ( 'NONE', ( #3453, #1257, #1882, #5394 ) ) ;
#1404=ADVANCED_FACE ( 'NONE', ( #2668, #4206, #6573, #4285, #6502, #1365 ), #3642, .T. ) ;
#1413=VERTEX_POINT ( 'NONE', #5442 ) ;
#1414=EDGE_CURVE ( 'NONE', #7258, #4994, #4883, .T. ) ;
#1417=FACE_BOUND ( 'NONE', #5353, .T. ) ;
#1421=ORIENTED_EDGE ( 'NONE', *, *, #6, .T. ) ;
#1422=VERTEX_POINT ( 'NONE', #2114 ) ;
#1434=EDGE_LOOP ( 'NONE', ( #5498, #6028, #3512, #7104 ) ) ;
#1437=VECTOR ( 'NONE', #433, 1000.000000000000000 ) ;
#1439=ORIENTED_EDGE ( 'NONE', *, *, #6730, .T. ) ;
#1441=ORIENTED_EDGE ( 'NONE', *, *, #3560, .T. ) ;
#1442=PLANE ( 'NONE',  #4244 ) ;
#1443=VECTOR ( 'NONE', #4126, 1000.000000000000000 ) ;
#1444=EDGE_CURVE ( 'NONE', #2259, #6037, #1625, .T. ) ;
#1448=CARTESIAN_POINT ( 'NONE',  ( 325.0000000000000000, 8.660254037844390851, 145.0000000000000284 ) ) ;
#1454=VECTOR ( 'NONE', #4253, 1000.000000000000000 ) ;
#1457=ORIENTED_EDGE ( 'NONE', *, *, #5359, .T. ) ;
#1458=DIRECTION ( 'NONE',  ( -0.000000000000000000, 0.000000000000000000, -1.000000000000000000 ) ) ;
#1459=CARTESIAN_POINT ( 'NONE',  ( 275.0000000000000000, 8.660254037844390851, 140.0000000000000000 ) ) ;
#1469=DIRECTION ( 'NONE',  ( 0.000000000000000000, 0.000000000000000000, 1.000000000000000000 ) ) ;
#1473=ORIENTED_EDGE ( 'NONE', *, *, #2995, .F. ) ;
#1474=DIRECTION ( 'NONE',  ( 0.000000000000000000, 1.000000000000000000, 0.000000000000000000 ) ) ;
#1475=VECTOR ( 'NONE', #2394, 1000.000000000000000 ) ;
#1481=AXIS2_PLACEMENT_3D ( 'NONE', #6686, #1583, #4957 ) ;
#1483=ORIENTED_EDGE ( 'NONE', *, *, #5965, .F. ) ;
#1485=ORIENTED_EDGE ( 'NONE', *, *, #3536, .T. ) ;
#1487=CARTESIAN_POINT ( 'NONE',  ( 195.0000000000000000, 8.660254037844390851, 139.9990000000000236 ) ) ;
#1490=AXIS2_PLACEMENT_3D ( 'NONE', #4896, #4987, #2126 ) ;
#1491=EDGE_LOOP ( 'NONE', ( #1473, #6420, #1799, #636 ) ) ;
#1493=EDGE_CURVE ( 'NONE', #4461, #4011, #6770, .T. ) ;
#1495=PLANE ( 'NONE',  #38 ) ;
#1496=FACE_OUTER_BOUND ( 'NONE', #5581, .T. ) ;
#1497=VECTOR ( 'NONE', #2553, 1000.000000000000000 ) ;
#1502=VERTEX_POINT ( 'NONE', #2705 ) ;
#1503=EDGE_CURVE ( 'NONE', #2165, #2018, #5078, .T. ) ;
#1505=LINE ( 'NONE', #5966, #133 ) ;
#1506=AXIS2_PLACEMENT_3D ( 'NONE', #4392, #5658, #5547 ) ;
#1507=FACE_OUTER_BOUND ( 'NONE', #4241, .T. ) ;
#1516=LINE ( 'NONE', #3249, #5156 ) ;
#1522=DIRECTION ( 'NONE',  ( -0.000000000000000000, -0.000000000000000000, 1.000000000000000000 ) ) ;
#1523=VERTEX_POINT ( 'NONE', #6807 ) ;
#1527=EDGE_CURVE ( 'NONE', #2818, #1325, #3372, .T. ) ;
#1532=DIRECTION ( 'NONE',  ( 0.000000000000000000, 0.000000000000000000, -1.000000000000000000 ) ) ;
#1534=CARTESIAN_POINT ( 'NONE',  ( 195.0000000000000000, -8.660254037844389075, 145.0000000000000284 ) ) ;
#1535=FACE_BOUND ( 'NONE', #697, .T. ) ;
#1538=VERTEX_POINT ( 'NONE', #6093 ) ;
#1543=CARTESIAN_POINT ( 'NONE',  ( 275.0000000000000000, 8.660254037844390851, 139.9990000000000236 ) ) ;
#1552=DIRECTION ( 'NONE',  ( -0.000000000000000000, 1.000000000000000000, -0.000000000000000000 ) ) ;
#1554=CARTESIAN_POINT ( 'NONE',  ( 4.999999999999999112, 8.660254037844390851, 140.0000000000000000 ) ) ;
#1558=ADVANCED_FACE ( 'NONE', ( #289 ), #3929, .F. ) ;
#1564=DIRECTION ( 'NONE',  ( 0.000000000000000000, -1.000000000000000000, 0.000000000000000000 ) ) ;
#1567=EDGE_CURVE ( 'NONE', #7307, #4268, #398, .T. ) ;
#1568=EDGE_LOOP ( 'NONE', ( #3636, #7115, #3421, #1201 ) ) ;
#1572=DIRECTION ( 'NONE',  ( -0.000000000000000000, 1.000000000000000000, -0.000000000000000000 ) ) ;
#1582=LINE ( 'NONE', #4953, #5915 ) ;
#1583=DIRECTION ( 'NONE',  ( -0.000000000000000000, 1.000000000000000000, -0.000000000000000000 ) ) ;
#1586=ORIENTED_EDGE ( 'NONE', *, *, #7280, .F. ) ;
#1588=LINE ( 'NONE', #6605, #5266 ) ;
#1589=CARTESIAN_POINT ( 'NONE',  ( 303.3333333333333144, -15.00000000000000000, 162.5000000000000853 ) ) ;
#1590=EDGE_CURVE ( 'NONE', #6398, #1084, #1036, .T. ) ;
#1593=DIRECTION ( 'NONE',  ( -0.000000000000000000, -0.000000000000000000, 1.000000000000000000 ) ) ;
#1596=VERTEX_POINT ( 'NONE', #2740 ) ;
#1598=VERTEX_POINT ( 'NONE', #2108 ) ;
#1604=CARTESIAN_POINT ( 'NONE',  ( 435.0000000000000568, 8.660254037844390851, 139.9990000000000236 ) ) ;
#1605=CARTESIAN_POINT ( 'NONE',  ( 53.33333333333330017, -20.00000000000000000, 162.5000000000000853 ) ) ;
#1613=EDGE_CURVE ( 'NONE', #1502, #2383, #6056, .T. ) ;
#1616=CARTESIAN_POINT ( 'NONE',  ( 53.33333333333330017, -20.00000000000000000, 159.8500000000001080 ) ) ;
#1618=VECTOR ( 'NONE', #2592, 1000.000000000000000 ) ;
#1619=LINE ( 'NONE', #645, #4087 ) ;
#1623=VECTOR ( 'NONE', #2260, 1000.000000000000000 ) ;
#1625=CIRCLE ( 'NONE', #5693, 2.649999999999985700 ) ;
#1626=ADVANCED_FACE ( 'NONE', ( #5179 ), #618, .F. ) ;
#1627=DIRECTION ( 'NONE',  ( -0.000000000000000000, 1.000000000000000000, 0.000000000000000000 ) ) ;
#1630=CARTESIAN_POINT ( 'NONE',  ( 4.999999999999999112, 8.660254037844390851, 145.0000000000000284 ) ) ;
#1636=AXIS2_PLACEMENT_3D ( 'NONE', #6819, #1158, #7338 ) ;
#1637=ORIENTED_EDGE ( 'NONE', *, *, #7141, .T. ) ;
#1639=DIRECTION ( 'NONE',  ( 0.000000000000000000, -0.000000000000000000, -1.000000000000000000 ) ) ;
#1642=ORIENTED_EDGE ( 'NONE', *, *, #5048, .F. ) ;
#1646=CARTESIAN_POINT ( 'NONE',  ( 84.99999999999998579, 8.660254037844390851, 139.9990000000000236 ) ) ;
#1649=DIRECTION ( 'NONE',  ( -0.000000000000000000, -0.000000000000000000, 1.000000000000000000 ) ) ;
#1651=ORIENTED_EDGE ( 'NONE', *, *, #5306, .F. ) ;
#1654=DIRECTION ( 'NONE',  ( -0.000000000000000000, 0.000000000000000000, 1.000000000000000000 ) ) ;
#1655=CARTESIAN_POINT ( 'NONE',  ( 53.33333333333330017, -14.99999999999999822, 162.5000000000000853 ) ) ;
#1658=CARTESIAN_POINT ( 'NONE',  ( 365.0000000000000000, 8.660254037844390851, 145.0000000000000284 ) ) ;
#1661=EDGE_CURVE ( 'NONE', #7340, #1770, #6652, .T. ) ;
#1662=EDGE_LOOP ( 'NONE', ( #6100, #5267, #1842, #3450 ) ) ;
#1664=DIRECTION ( 'NONE',  ( 0.000000000000000000, 0.000000000000000000, 1.000000000000000000 ) ) ;
#1666=FACE_BOUND ( 'NONE', #4720, .T. ) ;
#1669=EDGE_LOOP ( 'NONE', ( #4546, #3216, #1776, #6910 ) ) ;
#1674=ORIENTED_EDGE ( 'NONE', *, *, #5009, .T. ) ;
#1675=DIRECTION ( 'NONE',  ( 1.000000000000000000, 0.000000000000000000, 0.000000000000000000 ) ) ;
#1676=DIRECTION ( 'NONE',  ( 0.000000000000000000, -1.000000000000000000, 0.000000000000000000 ) ) ;
#1681=EDGE_LOOP ( 'NONE', ( #3263, #1966, #884, #6972 ) ) ;
#1682=DIRECTION ( 'NONE',  ( 1.000000000000000000, 0.000000000000000000, 0.000000000000000000 ) ) ;
#1683=VECTOR ( 'NONE', #2914, 1000.000000000000000 ) ;
#1684=CIRCLE ( 'NONE', #5868, 2.649999999999985700 ) ;
#1686=DIRECTION ( 'NONE',  ( -1.000000000000000000, 0.000000000000000000, -0.000000000000000000 ) ) ;
#1690=EDGE_CURVE ( 'NONE', #2383, #1502, #2328, .T. ) ;
#1691=ORIENTED_EDGE ( 'NONE', *, *, #6926, .T. ) ;
#1694=EDGE_LOOP ( 'NONE', ( #2131, #741, #3922, #2257 ) ) ;
#1698=CARTESIAN_POINT ( 'NONE',  ( 53.33333333333330017, -20.00000000000000000, 165.1500000000000625 ) ) ;
#1705=FACE_OUTER_BOUND ( 'NONE', #3662, .T. ) ;
#1706=VECTOR ( 'NONE', #7328, 1000.000000000000000 ) ;
#1710=EDGE_CURVE ( 'NONE', #3158, #6404, #5216, .T. ) ;
#1713=LINE ( 'NONE', #5614, #551 ) ;
#1714=CIRCLE ( 'NONE', #3743, 2.649999999999985700 ) ;
#1722=ORIENTED_EDGE ( 'NONE', *, *, #2701, .T. ) ;
#1724=CARTESIAN_POINT ( 'NONE',  ( 136.6666666666666288, -14.99999999999999822, 159.8500000000001080 ) ) ;
#1731=VERTEX_POINT ( 'NONE', #1459 ) ;
#1733=ADVANCED_FACE ( 'NONE', ( #1935 ), #3086, .F. ) ;
#1734=AXIS2_PLACEMENT_3D ( 'NONE', #528, #1256, #731 ) ;
#1737=DIRECTION ( 'NONE',  ( -0.000000000000000000, 1.000000000000000000, -0.000000000000000000 ) ) ;
#1742=ORIENTED_EDGE ( 'NONE', *, *, #2024, .T. ) ;
#1755=LINE ( 'NONE', #6793, #3009 ) ;
#1756=ORIENTED_EDGE ( 'NONE', *, *, #4834, .T. ) ;
#1758=DIRECTION ( 'NONE',  ( -1.000000000000000000, 0.000000000000000000, -0.000000000000000000 ) ) ;
#1766=CYLINDRICAL_SURFACE ( 'NONE', #5756, 2.649999999999985700 ) ;
#1768=EDGE_CURVE ( 'NONE', #7293, #1308, #315, .T. ) ;
#1770=VERTEX_POINT ( 'NONE', #6564 ) ;
#1775=FACE_OUTER_BOUND ( 'NONE', #519, .T. ) ;
#1776=ORIENTED_EDGE ( 'NONE', *, *, #4734, .F. ) ;
#1778=CARTESIAN_POINT ( 'NONE',  ( 45.00000000000000000, -8.660254037844389075, 139.9990000000000236 ) ) ;
#1779=ADVANCED_FACE ( 'NONE', ( #3014 ), #3738, .F. ) ;
#1782=VERTEX_POINT ( 'NONE', #239 ) ;
#1783=EDGE_CURVE ( 'NONE', #2951, #7258, #5967, .T. ) ;
#1785=DIRECTION ( 'NONE',  ( 0.000000000000000000, -1.000000000000000000, 0.000000000000000000 ) ) ;
#1786=DIRECTION ( 'NONE',  ( -0.000000000000000000, 0.000000000000000000, 1.000000000000000000 ) ) ;
#1787=CARTESIAN_POINT ( 'NONE',  ( -5.000000000000000888, -8.660254037844389075, 140.0000000000000000 ) ) ;
#1789=ORIENTED_EDGE ( 'NONE', *, *, #67, .T. ) ;
#1792=LINE ( 'NONE', #3547, #1443 ) ;
#1793=DIRECTION ( 'NONE',  ( 0.000000000000000000, -0.000000000000000000, -1.000000000000000000 ) ) ;
#1794=DIRECTION ( 'NONE',  ( -0.000000000000000000, 1.000000000000000000, -0.000000000000000000 ) ) ;
#1799=ORIENTED_EDGE ( 'NONE', *, *, #593, .F. ) ;
#1811=VECTOR ( 'NONE', #1305, 1000.000000000000000 ) ;
#1812=CARTESIAN_POINT ( 'NONE',  ( 155.0000000000000000, -8.660254037844389075, 145.0000000000000284 ) ) ;
#1817=CARTESIAN_POINT ( 'NONE',  ( 303.3333333333333144, -14.99999999999999822, 162.5000000000000853 ) ) ;
#1820=CARTESIAN_POINT ( 'NONE',  ( 155.0000000000000000, 8.660254037844390851, 145.0000000000000284 ) ) ;
#1822=ORIENTED_EDGE ( 'NONE', *, *, #368, .F. ) ;
#1825=PLANE ( 'NONE',  #1827 ) ;
#1827=AXIS2_PLACEMENT_3D ( 'NONE', #2939, #3660, #5880 ) ;
#1828=UNCERTAINTY_MEASURE_WITH_UNIT (LENGTH_MEASURE( 1.000000000000000082E-05 ), #2358, 'distance_accuracy_value', 'NONE');
#1829=ORIENTED_EDGE ( 'NONE', *, *, #4389, .F. ) ;
#1830=ORIENTED_EDGE ( 'NONE', *, *, #6194, .F. ) ;
#1831=CARTESIAN_POINT ( 'NONE',  ( 195.0000000000000000, -8.660254037844389075, 140.0000000000000000 ) ) ;
#1833=AXIS2_PLACEMENT_3D ( 'NONE', #4520, #6809, #6240 ) ;
#1837=CARTESIAN_POINT ( 'NONE',  ( 235.0000000000000000, -8.660254037844389075, 139.9990000000000236 ) ) ;
#1838=VECTOR ( 'NONE', #341, 1000.000000000000000 ) ;
#1842=ORIENTED_EDGE ( 'NONE', *, *, #7244, .F. ) ;
#1843=DIRECTION ( 'NONE',  ( 0.000000000000000000, 0.000000000000000000, -1.000000000000000000 ) ) ;
#1844=ORIENTED_EDGE ( 'NONE', *, *, #474, .T. ) ;
#1847=AXIS2_PLACEMENT_3D ( 'NONE', #554, #3871, #7250 ) ;
#1851=CARTESIAN_POINT ( 'NONE',  ( 124.9999999999999858, 8.660254037844390851, 139.9990000000000236 ) ) ;
#1856=ORIENTED_EDGE ( 'NONE', *, *, #6926, .F. ) ;
#1859=DIRECTION ( 'NONE',  ( -0.000000000000000000, 1.000000000000000000, -0.000000000000000000 ) ) ;
#1862=ORIENTED_EDGE ( 'NONE', *, *, #6060, .T. ) ;
#1865=ORIENTED_EDGE ( 'NONE', *, *, #2024, .F. ) ;
#1868=DIRECTION ( 'NONE',  ( -1.000000000000000000, -0.000000000000000000, -0.000000000000000000 ) ) ;
#1869=CARTESIAN_POINT ( 'NONE',  ( 164.9999999999999716, 8.660254037844390851, 140.0000000000000000 ) ) ;
#1872=EDGE_CURVE ( 'NONE', #932, #1873, #2097, .T. ) ;
#1873=VERTEX_POINT ( 'NONE', #3860 ) ;
#1874=ORIENTED_EDGE ( 'NONE', *, *, #6455, .F. ) ;
#1876=DIRECTION ( 'NONE',  ( 0.000000000000000000, 0.000000000000000000, -1.000000000000000000 ) ) ;
#1877=EDGE_LOOP ( 'NONE', ( #3340, #747, #5135, #1756 ) ) ;
#1881=CARTESIAN_POINT ( 'NONE',  ( 164.9999999999999716, 8.660254037844390851, 140.0000000000000000 ) ) ;
#1882=ORIENTED_EDGE ( 'NONE', *, *, #4305, .F. ) ;
#1883=CARTESIAN_POINT ( 'NONE',  ( 136.6666666666666288, -20.00000000000000000, 165.1500000000000625 ) ) ;
#1884=VERTEX_POINT ( 'NONE', #4463 ) ;
#1890=EDGE_LOOP ( 'NONE', ( #1789, #7069, #4617, #1035 ) ) ;
#1891=LINE ( 'NONE', #6377, #4105 ) ;
#1892=ORIENTED_EDGE ( 'NONE', *, *, #652, .T. ) ;
#1893=EDGE_LOOP ( 'NONE', ( #5939, #5620, #4167, #1439 ) ) ;
#1899=ADVANCED_FACE ( 'NONE', ( #1507 ), #3288, .F. ) ;
#1906=DIRECTION ( 'NONE',  ( -0.000000000000000000, -0.000000000000000000, -1.000000000000000000 ) ) ;
#1907=EDGE_LOOP ( 'NONE', ( #2895, #322, #5015, #3092 ) ) ;
#1919=EDGE_CURVE ( 'NONE', #5019, #3377, #675, .T. ) ;
#1920=AXIS2_PLACEMENT_3D ( 'NONE', #6002, #5549, #2011 ) ;
#1924=DIRECTION ( 'NONE',  ( -1.000000000000000000, -0.000000000000000000, -0.000000000000000000 ) ) ;
#1925=EDGE_CURVE ( 'NONE', #6714, #1367, #6083, .T. ) ;
#1929=PRODUCT_DEFINITION_SHAPE ( 'NONE', 'NONE',  #2657 ) ;
#1933=VERTEX_POINT ( 'NONE', #945 ) ;
#1934=PLANE ( 'NONE',  #142 ) ;
#1935=FACE_OUTER_BOUND ( 'NONE', #4057, .T. ) ;
#1939=VECTOR ( 'NONE', #5291, 1000.000000000000000 ) ;
#1941=ADVANCED_FACE ( 'NONE', ( #2805 ), #7195, .F. ) ;
#1942=CARTESIAN_POINT ( 'NONE',  ( 365.0000000000000000, -8.660254037844389075, 139.9990000000000236 ) ) ;
#1948=LINE ( 'NONE', #1361, #3023 ) ;
#1957=VECTOR ( 'NONE', #464, 1000.000000000000000 ) ;
#1963=AXIS2_PLACEMENT_3D ( 'NONE', #2294, #628, #5829 ) ;
#1964=EDGE_CURVE ( 'NONE', #1538, #767, #6370, .T. ) ;
#1965=AXIS2_PLACEMENT_3D ( 'NONE', #588, #5246, #6423 ) ;
#1966=ORIENTED_EDGE ( 'NONE', *, *, #2368, .F. ) ;
#1969=CARTESIAN_POINT ( 'NONE',  ( -30.00000000000002842, -20.00000000000000000, 180.0000000000000284 ) ) ;
#1971=AXIS2_PLACEMENT_3D ( 'NONE', #2233, #6461, #1843 ) ;
#1972=VERTEX_POINT ( 'NONE', #6831 ) ;
#1974=EDGE_LOOP ( 'NONE', ( #5699, #7205, #5381, #687 ) ) ;
#1975=AXIS2_PLACEMENT_3D ( 'NONE', #1192, #4098, #4633 ) ;
#1984=ORIENTED_EDGE ( 'NONE', *, *, #1590, .F. ) ;
#1985=LINE ( 'NONE', #4024, #5867 ) ;
#1986=CARTESIAN_POINT ( 'NONE',  ( -30.00000000000002842, 15.00000000000000000, 145.0000000000000284 ) ) ;
#1988=ADVANCED_FACE ( 'NONE', ( #934 ), #5169, .F. ) ;
#1990=ORIENTED_EDGE ( 'NONE', *, *, #1240, .T. ) ;
#1991=ORIENTED_EDGE ( 'NONE', *, *, #2112, .F. ) ;
#1996=PLANE ( 'NONE',  #2421 ) ;
#2003=EDGE_CURVE ( 'NONE', #84, #4019, #3503, .T. ) ;
#2007=VERTEX_POINT ( 'NONE', #1724 ) ;
#2011=DIRECTION ( 'NONE',  ( 0.000000000000000000, -0.000000000000000000, -1.000000000000000000 ) ) ;
#2018=VERTEX_POINT ( 'NONE', #6933 ) ;
#2022=CARTESIAN_POINT ( 'NONE',  ( 45.00000000000000000, 8.660254037844390851, 140.0000000000000000 ) ) ;
#2024=EDGE_CURVE ( 'NONE', #2259, #6322, #4041, .T. ) ;
#2032=DIRECTION ( 'NONE',  ( -0.000000000000000000, 1.000000000000000000, -0.000000000000000000 ) ) ;
#2034=EDGE_LOOP ( 'NONE', ( #875, #1722, #21, #4239 ) ) ;
#2039=CARTESIAN_POINT ( 'NONE',  ( 435.0000000000000568, 8.660254037844390851, 139.9990000000000236 ) ) ;
#2043=CARTESIAN_POINT ( 'NONE',  ( 205.0000000000000284, 8.660254037844390851, 140.0000000000000000 ) ) ;
#2044=VECTOR ( 'NONE', #3739, 1000.000000000000000 ) ;
#2045=VECTOR ( 'NONE', #6550, 1000.000000000000000 ) ;
#2049=LINE ( 'NONE', #2095, #2266 ) ;
#2051=DIRECTION ( 'NONE',  ( -0.000000000000000000, 1.000000000000000000, -0.000000000000000000 ) ) ;
#2062=VERTEX_POINT ( 'NONE', #16 ) ;
#2066=SURFACE_STYLE_USAGE ( .BOTH. , #4245 ) ;
#2067=CARTESIAN_POINT ( 'NONE',  ( 395.0000000000000000, 8.660254037844390851, 139.9990000000000236 ) ) ;
#2071=VECTOR ( 'NONE', #2769, 1000.000000000000000 ) ;
#2074=EDGE_LOOP ( 'NONE', ( #6542, #4949, #5458, #606 ) ) ;
#2076=DIRECTION ( 'NONE',  ( -1.000000000000000000, 0.000000000000000000, 0.000000000000000000 ) ) ;
#2077=CIRCLE ( 'NONE', #4596, 2.649999999999985700 ) ;
#2078=DIRECTION ( 'NONE',  ( 0.000000000000000000, 0.000000000000000000, 1.000000000000000000 ) ) ;
#2084=CARTESIAN_POINT ( 'NONE',  ( 195.0000000000000000, 8.660254037844390851, 139.9990000000000236 ) ) ;
#2085=ADVANCED_FACE ( 'NONE', ( #4572 ), #6865, .F. ) ;
#2086=DIRECTION ( 'NONE',  ( 0.000000000000000000, -1.000000000000000000, 0.000000000000000000 ) ) ;
#2087=DIRECTION ( 'NONE',  ( -1.000000000000000000, 0.000000000000000000, -0.000000000000000000 ) ) ;
#2095=CARTESIAN_POINT ( 'NONE',  ( 395.0000000000000000, -8.660254037844389075, 145.0000000000000284 ) ) ;
#2097=LINE ( 'NONE', #2134, #3644 ) ;
#2099=CARTESIAN_POINT ( 'NONE',  ( 4.999999999999999112, 8.660254037844390851, 139.9990000000000236 ) ) ;
#2101=EDGE_CURVE ( 'NONE', #7234, #1078, #644, .T. ) ;
#2105=AXIS2_PLACEMENT_3D ( 'NONE', #4891, #2032, #258 ) ;
#2108=CARTESIAN_POINT ( 'NONE',  ( 45.00000000000000000, -8.660254037844389075, 145.0000000000000284 ) ) ;
#2109=CARTESIAN_POINT ( 'NONE',  ( 435.0000000000000568, 8.660254037844390851, 145.0000000000000284 ) ) ;
#2112=EDGE_CURVE ( 'NONE', #7144, #5826, #2965, .T. ) ;
#2114=CARTESIAN_POINT ( 'NONE',  ( 435.0000000000000568, 8.660254037844390851, 145.0000000000000284 ) ) ;
#2118=EDGE_LOOP ( 'NONE', ( #3607, #6919, #1485, #6157 ) ) ;
#2119=CARTESIAN_POINT ( 'NONE',  ( 355.0000000000000000, -8.660254037844389075, 139.9990000000000236 ) ) ;
#2121=CARTESIAN_POINT ( 'NONE',  ( 435.0000000000000568, 8.660254037844390851, 140.0000000000000000 ) ) ;
#2122=ORIENTED_EDGE ( 'NONE', *, *, #1493, .F. ) ;
#2125=LINE ( 'NONE', #6585, #5517 ) ;
#2126=DIRECTION ( 'NONE',  ( 0.000000000000000000, 0.000000000000000000, -1.000000000000000000 ) ) ;
#2130=ADVANCED_FACE ( 'NONE', ( #2413 ), #5897, .F. ) ;
#2131=ORIENTED_EDGE ( 'NONE', *, *, #3639, .F. ) ;
#2134=CARTESIAN_POINT ( 'NONE',  ( 195.0000000000000000, 8.660254037844390851, 140.0000000000000000 ) ) ;
#2136=DIRECTION ( 'NONE',  ( -0.000000000000000000, -0.000000000000000000, 1.000000000000000000 ) ) ;
#2141=LINE ( 'NONE', #4434, #730 ) ;
#2148=ORIENTED_EDGE ( 'NONE', *, *, #2991, .F. ) ;
#2151=ORIENTED_EDGE ( 'NONE', *, *, #5251, .T. ) ;
#2155=CARTESIAN_POINT ( 'NONE',  ( 35.00000000000000000, 8.660254037844390851, 139.9990000000000236 ) ) ;
#2157=VERTEX_POINT ( 'NONE', #1319 ) ;
#2161=CARTESIAN_POINT ( 'NONE',  ( 470.0000000000000000, 0.000000000000000000, 145.0000000000000284 ) ) ;
#2165=VERTEX_POINT ( 'NONE', #3558 ) ;
#2168=FACE_OUTER_BOUND ( 'NONE', #5066, .T. ) ;
#2176=CARTESIAN_POINT ( 'NONE',  ( 195.0000000000000000, 8.660254037844390851, 145.0000000000000284 ) ) ;
#2179=EDGE_CURVE ( 'NONE', #3697, #2491, #4168, .T. ) ;
#2180=FACE_OUTER_BOUND ( 'NONE', #3593, .T. ) ;
#2182=CIRCLE ( 'NONE', #525, 2.649999999999985700 ) ;
#2183=ORIENTED_EDGE ( 'NONE', *, *, #3248, .F. ) ;
#2185=VERTEX_POINT ( 'NONE', #5859 ) ;
#2186=LINE ( 'NONE', #3842, #1034 ) ;
#2191=LINE ( 'NONE', #2667, #5220 ) ;
#2192=ADVANCED_FACE ( 'NONE', ( #7026 ), #2755, .F. ) ;
#2199=EDGE_CURVE ( 'NONE', #4599, #3059, #3486, .T. ) ;
#2202=LINE ( 'NONE', #4501, #1138 ) ;
#2204=ORIENTED_EDGE ( 'NONE', *, *, #1049, .T. ) ;
#2205=VERTEX_POINT ( 'NONE', #5055 ) ;
#2208=VECTOR ( 'NONE', #5866, 1000.000000000000000 ) ;
#2210=DIRECTION ( 'NONE',  ( -1.000000000000000000, 0.000000000000000000, 0.000000000000000000 ) ) ;
#2220=DIRECTION ( 'NONE',  ( -0.000000000000000000, 1.000000000000000000, -0.000000000000000000 ) ) ;
#2225=EDGE_CURVE ( 'NONE', #2205, #3050, #666, .T. ) ;
#2227=VECTOR ( 'NONE', #7179, 1000.000000000000000 ) ;
#2228=ORIENTED_EDGE ( 'NONE', *, *, #819, .F. ) ;
#2232=ORIENTED_EDGE ( 'NONE', *, *, #1293, .F. ) ;
#2233=CARTESIAN_POINT ( 'NONE',  ( 325.0000000000000000, 8.660254037844390851, 139.9990000000000236 ) ) ;
#2234=EDGE_CURVE ( 'NONE', #4657, #3206, #7099, .T. ) ;
#2237=ADVANCED_FACE ( 'NONE', ( #6218 ), #2436, .F. ) ;
#2241=ORIENTED_EDGE ( 'NONE', *, *, #4287, .F. ) ;
#2245=LINE ( 'NONE', #3978, #3480 ) ;
#2249=VERTEX_POINT ( 'NONE', #106 ) ;
#2252=DIRECTION ( 'NONE',  ( 0.000000000000000000, 0.000000000000000000, -1.000000000000000000 ) ) ;
#2257=ORIENTED_EDGE ( 'NONE', *, *, #4935, .T. ) ;
#2259=VERTEX_POINT ( 'NONE', #6946 ) ;
#2260=DIRECTION ( 'NONE',  ( -0.000000000000000000, -0.000000000000000000, 1.000000000000000000 ) ) ;
#2263=ORIENTED_EDGE ( 'NONE', *, *, #1115, .T. ) ;
#2265=LINE ( 'NONE', #3969, #4014 ) ;
#2266=VECTOR ( 'NONE', #6681, 1000.000000000000000 ) ;
#2271=LINE ( 'NONE', #5733, #2896 ) ;
#2272=EDGE_CURVE ( 'NONE', #1308, #2725, #4840, .T. ) ;
#2279=ORIENTED_EDGE ( 'NONE', *, *, #4837, .T. ) ;
#2280=DIRECTION ( 'NONE',  ( -1.000000000000000000, 0.000000000000000000, 0.000000000000000000 ) ) ;
#2285=LINE ( 'NONE', #5180, #1683 ) ;
#2286=FACE_BOUND ( 'NONE', #6470, .T. ) ;
#2291=ORIENTED_EDGE ( 'NONE', *, *, #6513, .F. ) ;
#2294=CARTESIAN_POINT ( 'NONE',  ( 0.000000000000000000, 0.000000000000000000, 0.000000000000000000 ) ) ;
#2300=DIRECTION ( 'NONE',  ( -0.000000000000000000, 1.000000000000000000, 0.000000000000000000 ) ) ;
#2312=LINE ( 'NONE', #3470, #268 ) ;
#2313=DIRECTION ( 'NONE',  ( 0.000000000000000000, -1.000000000000000000, 0.000000000000000000 ) ) ;
#2316=( GEOMETRIC_REPRESENTATION_CONTEXT ( 3 ) GLOBAL_UNCERTAINTY_ASSIGNED_CONTEXT ( ( #772 ) ) GLOBAL_UNIT_ASSIGNED_CONTEXT ( ( #4843, #6656, #7134 ) ) REPRESENTATION_CONTEXT ( 'NONE', 'WORKASPACE' ) );
#2317=EDGE_LOOP ( 'NONE', ( #2854, #4750, #4399, #2393 ) ) ;
#2323=LINE ( 'NONE', #6940, #6721 ) ;
#2327=LINE ( 'NONE', #4627, #6023 ) ;
#2328=CIRCLE ( 'NONE', #3030, 2.649999999999985700 ) ;
#2331=ORIENTED_EDGE ( 'NONE', *, *, #234, .F. ) ;
#2333=VECTOR ( 'NONE', #5204, 1000.000000000000000 ) ;
#2335=CARTESIAN_POINT ( 'NONE',  ( 395.0000000000000000, -8.660254037844389075, 139.9990000000000236 ) ) ;
#2338=DIRECTION ( 'NONE',  ( 0.000000000000000000, 1.000000000000000000, 0.000000000000000000 ) ) ;
#2341=CYLINDRICAL_SURFACE ( 'NONE', #3215, 2.649999999999985700 ) ;
#2353=PLANE ( 'NONE',  #5996 ) ;
#2354=DIRECTION ( 'NONE',  ( -0.000000000000000000, -0.000000000000000000, 1.000000000000000000 ) ) ;
#2355=CARTESIAN_POINT ( 'NONE',  ( -30.00000000000002842, -20.00000000000000000, 180.0000000000000284 ) ) ;
#2356=FACE_BOUND ( 'NONE', #1491, .T. ) ;
#2358=( LENGTH_UNIT ( ) NAMED_UNIT ( * ) SI_UNIT ( .MILLI., .METRE. ) );
#2361=CARTESIAN_POINT ( 'NONE',  ( 114.9999999999999858, 8.660254037844390851, 145.0000000000000284 ) ) ;
#2365=EDGE_CURVE ( 'NONE', #818, #2818, #1948, .T. ) ;
#2368=EDGE_CURVE ( 'NONE', #7046, #2165, #246, .T. ) ;
#2370=LINE ( 'NONE', #1265, #4700 ) ;
#2374=DIRECTION ( 'NONE',  ( -0.000000000000000000, 1.000000000000000000, 0.000000000000000000 ) ) ;
#2380=ORIENTED_EDGE ( 'NONE', *, *, #1222, .T. ) ;
#2381=DIRECTION ( 'NONE',  ( 0.000000000000000000, 0.000000000000000000, 1.000000000000000000 ) ) ;
#2382=AXIS2_PLACEMENT_3D ( 'NONE', #5081, #6916, #3416 ) ;
#2383=VERTEX_POINT ( 'NONE', #6606 ) ;
#2390=AXIS2_PLACEMENT_3D ( 'NONE', #5147, #1627, #5630 ) ;
#2393=ORIENTED_EDGE ( 'NONE', *, *, #319, .F. ) ;
#2394=DIRECTION ( 'NONE',  ( 0.000000000000000000, 1.000000000000000000, 0.000000000000000000 ) ) ;
#2396=EDGE_CURVE ( 'NONE', #7307, #3059, #4878, .T. ) ;
#2397=CARTESIAN_POINT ( 'NONE',  ( 275.0000000000000000, -8.660254037844389075, 145.0000000000000284 ) ) ;
#2402=CARTESIAN_POINT ( 'NONE',  ( 235.0000000000000000, -8.660254037844389075, 145.0000000000000284 ) ) ;
#2403=EDGE_CURVE ( 'NONE', #1884, #4228, #3792, .T. ) ;
#2405=ORIENTED_EDGE ( 'NONE', *, *, #3223, .F. ) ;
#2412=CARTESIAN_POINT ( 'NONE',  ( 114.9999999999999858, -8.660254037844389075, 139.9990000000000236 ) ) ;
#2413=FACE_OUTER_BOUND ( 'NONE', #3179, .T. ) ;
#2414=FACE_OUTER_BOUND ( 'NONE', #1681, .T. ) ;
#2420=CARTESIAN_POINT ( 'NONE',  ( 164.9999999999999716, -8.660254037844389075, 145.0000000000000284 ) ) ;
#2421=AXIS2_PLACEMENT_3D ( 'NONE', #2155, #4447, #3768 ) ;
#2424=ORIENTED_EDGE ( 'NONE', *, *, #6184, .F. ) ;
#2425=DIRECTION ( 'NONE',  ( 0.000000000000000000, -1.000000000000000000, 0.000000000000000000 ) ) ;
#2427=CIRCLE ( 'NONE', #4823, 2.649999999999985700 ) ;
#2429=DIRECTION ( 'NONE',  ( 1.000000000000000000, 0.000000000000000000, 0.000000000000000000 ) ) ;
#2430=DIRECTION ( 'NONE',  ( 0.000000000000000000, -1.000000000000000000, 0.000000000000000000 ) ) ;
#2431=CARTESIAN_POINT ( 'NONE',  ( 395.0000000000000000, 8.660254037844390851, 139.9990000000000236 ) ) ;
#2436=PLANE ( 'NONE',  #59 ) ;
#2444=DIRECTION ( 'NONE',  ( -0.000000000000000000, -0.000000000000000000, 1.000000000000000000 ) ) ;
#2445=VECTOR ( 'NONE', #5726, 1000.000000000000000 ) ;
#2448=CARTESIAN_POINT ( 'NONE',  ( 245.0000000000000000, 8.660254037844390851, 145.0000000000000284 ) ) ;
#2449=ORIENTED_EDGE ( 'NONE', *, *, #2603, .T. ) ;
#2464=CARTESIAN_POINT ( 'NONE',  ( 124.9999999999999858, -8.660254037844389075, 140.0000000000000000 ) ) ;
#2476=EDGE_LOOP ( 'NONE', ( #969, #6838 ) ) ;
#2477=ORIENTED_EDGE ( 'NONE', *, *, #3702, .F. ) ;
#2478=DIRECTION ( 'NONE',  ( -1.000000000000000000, 0.000000000000000000, -0.000000000000000000 ) ) ;
#2481=ORIENTED_EDGE ( 'NONE', *, *, #2112, .T. ) ;
#2482=DIRECTION ( 'NONE',  ( -0.000000000000000000, 1.000000000000000000, -0.000000000000000000 ) ) ;
#2485=DIRECTION ( 'NONE',  ( -0.000000000000000000, 1.000000000000000000, -0.000000000000000000 ) ) ;
#2490=VECTOR ( 'NONE', #643, 1000.000000000000000 ) ;
#2491=VERTEX_POINT ( 'NONE', #3127 ) ;
#2493=DIRECTION ( 'NONE',  ( -1.000000000000000000, 0.000000000000000000, 0.000000000000000000 ) ) ;
#2496=DIRECTION ( 'NONE',  ( 1.000000000000000000, 0.000000000000000000, 0.000000000000000000 ) ) ;
#2501=VECTOR ( 'NONE', #5149, 1000.000000000000000 ) ;
#2504=DIRECTION ( 'NONE',  ( -0.000000000000000000, -0.000000000000000000, 1.000000000000000000 ) ) ;
#2506=( LENGTH_UNIT ( ) NAMED_UNIT ( * ) SI_UNIT ( .MILLI., .METRE. ) );
#2511=CARTESIAN_POINT ( 'NONE',  ( 124.9999999999999858, 8.660254037844390851, 140.0000000000000000 ) ) ;
#2515=CARTESIAN_POINT ( 'NONE',  ( 245.0000000000000000, 8.660254037844390851, 140.0000000000000000 ) ) ;
#2516=LINE ( 'NONE', #4931, #3294 ) ;
#2520=LINE ( 'NONE', #2084, #4689 ) ;
#2534=PRODUCT_DEFINITION_FORMATION_WITH_SPECIFIED_SOURCE ( 'ANY', '', #4155, .NOT_KNOWN. ) ;
#2544=EDGE_LOOP ( 'NONE', ( #5998, #3659, #458, #5612 ) ) ;
#2549=ADVANCED_FACE ( 'NONE', ( #4430 ), #2737, .F. ) ;
#2553=DIRECTION ( 'NONE',  ( 0.000000000000000000, -1.000000000000000000, 0.000000000000000000 ) ) ;
#2562=CARTESIAN_POINT ( 'NONE',  ( 355.0000000000000000, 8.660254037844390851, 145.0000000000000284 ) ) ;
#2567=ORIENTED_EDGE ( 'NONE', *, *, #1306, .F. ) ;
#2568=VECTOR ( 'NONE', #4068, 1000.000000000000000 ) ;
#2572=CARTESIAN_POINT ( 'NONE',  ( 114.9999999999999858, 8.660254037844390851, 139.9990000000000236 ) ) ;
#2573=CARTESIAN_POINT ( 'NONE',  ( -30.00000000000002842, -15.00000000000000000, 180.0000000000000284 ) ) ;
#2574=DIRECTION ( 'NONE',  ( -0.000000000000000000, 1.000000000000000000, -0.000000000000000000 ) ) ;
#2577=LINE ( 'NONE', #5971, #6637 ) ;
#2582=ORIENTED_EDGE ( 'NONE', *, *, #5293, .T. ) ;
#2584=ADVANCED_FACE ( 'NONE', ( #1033 ), #3246, .F. ) ;
#2586=EDGE_CURVE ( 'NONE', #5826, #3826, #990, .T. ) ;
#2587=CARTESIAN_POINT ( 'NONE',  ( 35.00000000000000000, -8.660254037844389075, 140.0000000000000000 ) ) ;
#2588=ORIENTED_EDGE ( 'NONE', *, *, #701, .T. ) ;
#2592=DIRECTION ( 'NONE',  ( 0.000000000000000000, -1.000000000000000000, 0.000000000000000000 ) ) ;
#2596=ORIENTED_EDGE ( 'NONE', *, *, #2396, .F. ) ;
#2603=EDGE_CURVE ( 'NONE', #6334, #7307, #4513, .T. ) ;
#2604=ORIENTED_EDGE ( 'NONE', *, *, #7280, .T. ) ;
#2607=ORIENTED_EDGE ( 'NONE', *, *, #5953, .T. ) ;
#2611=DIRECTION ( 'NONE',  ( -0.000000000000000000, -0.000000000000000000, 1.000000000000000000 ) ) ;
#2621=VECTOR ( 'NONE', #3085, 1000.000000000000000 ) ;
#2625=AXIS2_PLACEMENT_3D ( 'NONE', #5116, #4582, #617 ) ;
#2632=VECTOR ( 'NONE', #2493, 1000.000000000000000 ) ;
#2637=VECTOR ( 'NONE', #2766, 1000.000000000000000 ) ;
#2640=LINE ( 'NONE', #4381, #1838 ) ;
#2642=ORIENTED_EDGE ( 'NONE', *, *, #4199, .T. ) ;
#2645=ORIENTED_EDGE ( 'NONE', *, *, #24, .F. ) ;
#2653=DIRECTION ( 'NONE',  ( 0.000000000000000000, 0.000000000000000000, -1.000000000000000000 ) ) ;
#2654=AXIS2_PLACEMENT_3D ( 'NONE', #6659, #6774, #327 ) ;
#2656=DIRECTION ( 'NONE',  ( 0.000000000000000000, 0.000000000000000000, 1.000000000000000000 ) ) ;
#2657=PRODUCT_DEFINITION ( 'UNKNOWN', '', #2534, #6593 ) ;
#2658=ORIENTED_EDGE ( 'NONE', *, *, #1768, .T. ) ;
#2661=VECTOR ( 'NONE', #4131, 1000.000000000000000 ) ;
#2667=CARTESIAN_POINT ( 'NONE',  ( 35.00000000000000000, -8.660254037844389075, 140.0000000000000000 ) ) ;
#2668=FACE_BOUND ( 'NONE', #615, .T. ) ;
#2669=VECTOR ( 'NONE', #3356, 1000.000000000000000 ) ;
#2672=ORIENTED_EDGE ( 'NONE', *, *, #3223, .T. ) ;
#2676=VECTOR ( 'NONE', #986, 1000.000000000000000 ) ;
#2683=LINE ( 'NONE', #5020, #1223 ) ;
#2684=FACE_OUTER_BOUND ( 'NONE', #1694, .T. ) ;
#2688=VECTOR ( 'NONE', #2354, 1000.000000000000000 ) ;
#2701=EDGE_CURVE ( 'NONE', #767, #4657, #6232, .T. ) ;
#2704=DIRECTION ( 'NONE',  ( -0.000000000000000000, 1.000000000000000000, 0.000000000000000000 ) ) ;
#2705=CARTESIAN_POINT ( 'NONE',  ( 386.6666666666666288, -20.00000000000000000, 165.1500000000000625 ) ) ;
#2707=CARTESIAN_POINT ( 'NONE',  ( 315.0000000000000568, 8.660254037844390851, 145.0000000000000284 ) ) ;
#2711=VERTEX_POINT ( 'NONE', #6271 ) ;
#2721=EDGE_CURVE ( 'NONE', #6469, #6561, #2186, .T. ) ;
#2725=VERTEX_POINT ( 'NONE', #22 ) ;
#2726=CARTESIAN_POINT ( 'NONE',  ( 4.999999999999999112, 8.660254037844390851, 139.9990000000000236 ) ) ;
#2728=EDGE_CURVE ( 'NONE', #6875, #3397, #538, .T. ) ;
#2729=ORIENTED_EDGE ( 'NONE', *, *, #4854, .T. ) ;
#2735=EDGE_CURVE ( 'NONE', #4758, #4011, #509, .T. ) ;
#2737=PLANE ( 'NONE',  #6273 ) ;
#2740=CARTESIAN_POINT ( 'NONE',  ( 219.9999999999999716, -14.99999999999999822, 165.1500000000000625 ) ) ;
#2745=ORIENTED_EDGE ( 'NONE', *, *, #1613, .T. ) ;
#2750=ADVANCED_FACE ( 'NONE', ( #1101 ), #1825, .F. ) ;
#2753=DIRECTION ( 'NONE',  ( -0.000000000000000000, -0.000000000000000000, 1.000000000000000000 ) ) ;
#2754=ORIENTED_EDGE ( 'NONE', *, *, #6883, .F. ) ;
#2755=PLANE ( 'NONE',  #1734 ) ;
#2757=DIRECTION ( 'NONE',  ( -1.000000000000000000, 0.000000000000000000, 0.000000000000000000 ) ) ;
#2765=DIRECTION ( 'NONE',  ( -1.000000000000000000, 0.000000000000000000, 0.000000000000000000 ) ) ;
#2766=DIRECTION ( 'NONE',  ( -1.000000000000000000, 0.000000000000000000, 0.000000000000000000 ) ) ;
#2769=DIRECTION ( 'NONE',  ( -1.000000000000000000, -0.000000000000000000, -0.000000000000000000 ) ) ;
#2777=FACE_BOUND ( 'NONE', #963, .T. ) ;
#2778=AXIS2_PLACEMENT_3D ( 'NONE', #6284, #5783, #6349 ) ;
#2781=AXIS2_PLACEMENT_3D ( 'NONE', #1837, #5823, #1314 ) ;
#2787=LINE ( 'NONE', #5051, #7118 ) ;
#2789=VECTOR ( 'NONE', #4641, 1000.000000000000000 ) ;
#2791=EDGE_CURVE ( 'NONE', #6671, #7155, #1341, .T. ) ;
#2796=LINE ( 'NONE', #2827, #4704 ) ;
#2797=CARTESIAN_POINT ( 'NONE',  ( 386.6666666666666288, -14.99999999999999822, 162.5000000000000853 ) ) ;
#2801=CARTESIAN_POINT ( 'NONE',  ( 155.0000000000000000, 8.660254037844390851, 140.0000000000000000 ) ) ;
#2804=DIRECTION ( 'NONE',  ( -1.000000000000000000, 0.000000000000000000, 0.000000000000000000 ) ) ;
#2805=FACE_OUTER_BOUND ( 'NONE', #4089, .T. ) ;
#2808=DIRECTION ( 'NONE',  ( 1.000000000000000000, 0.000000000000000000, 0.000000000000000000 ) ) ;
#2813=CARTESIAN_POINT ( 'NONE',  ( 235.0000000000000000, 8.660254037844390851, 145.0000000000000284 ) ) ;
#2815=EDGE_CURVE ( 'NONE', #6064, #2249, #1891, .T. ) ;
#2818=VERTEX_POINT ( 'NONE', #2420 ) ;
#2820=AXIS2_PLACEMENT_3D ( 'NONE', #1605, #3925, #5574 ) ;
#2825=CARTESIAN_POINT ( 'NONE',  ( 435.0000000000000568, -8.660254037844389075, 140.0000000000000000 ) ) ;
#2826=VERTEX_POINT ( 'NONE', #4680 ) ;
#2827=CARTESIAN_POINT ( 'NONE',  ( 355.0000000000000000, 8.660254037844390851, 140.0000000000000000 ) ) ;
#2831=ORIENTED_EDGE ( 'NONE', *, *, #2179, .T. ) ;
#2833=AXIS2_PLACEMENT_3D ( 'NONE', #3117, #4761, #5388 ) ;
#2834=ORIENTED_EDGE ( 'NONE', *, *, #7031, .F. ) ;
#2840=EDGE_CURVE ( 'NONE', #224, #2007, #2182, .T. ) ;
#2843=EDGE_LOOP ( 'NONE', ( #886, #2263, #6993, #7228 ) ) ;
#2844=FACE_BOUND ( 'NONE', #6308, .T. ) ;
#2845=DIRECTION ( 'NONE',  ( 0.000000000000000000, 0.000000000000000000, 1.000000000000000000 ) ) ;
#2846=DIRECTION ( 'NONE',  ( 0.000000000000000000, 0.000000000000000000, 1.000000000000000000 ) ) ;
#2849=ORIENTED_EDGE ( 'NONE', *, *, #2586, .F. ) ;
#2854=ORIENTED_EDGE ( 'NONE', *, *, #1014, .F. ) ;
#2861=CIRCLE ( 'NONE', #2382, 2.649999999999985700 ) ;
#2864=EDGE_CURVE ( 'NONE', #828, #224, #5279, .T. ) ;
#2866=DIRECTION ( 'NONE',  ( -0.000000000000000000, 1.000000000000000000, -0.000000000000000000 ) ) ;
#2869=CARTESIAN_POINT ( 'NONE',  ( 303.3333333333333144, -14.99999999999999822, 165.1500000000000625 ) ) ;
#2875=FACE_OUTER_BOUND ( 'NONE', #4066, .T. ) ;
#2876=CARTESIAN_POINT ( 'NONE',  ( 275.0000000000000000, -8.660254037844389075, 139.9990000000000236 ) ) ;
#2879=VECTOR ( 'NONE', #1859, 1000.000000000000000 ) ;
#2882=ORIENTED_EDGE ( 'NONE', *, *, #3341, .T. ) ;
#2895=ORIENTED_EDGE ( 'NONE', *, *, #5380, .T. ) ;
#2896=VECTOR ( 'NONE', #5062, 1000.000000000000000 ) ;
#2898=FACE_OUTER_BOUND ( 'NONE', #2034, .T. ) ;
#2899=CARTESIAN_POINT ( 'NONE',  ( 235.0000000000000000, -8.660254037844389075, 140.0000000000000000 ) ) ;
#2901=DIRECTION ( 'NONE',  ( 0.000000000000000000, -1.000000000000000000, 0.000000000000000000 ) ) ;
#2907=EDGE_CURVE ( 'NONE', #4971, #6875, #3159, .T. ) ;
#2911=VECTOR ( 'NONE', #1264, 1000.000000000000000 ) ;
#2912=FACE_OUTER_BOUND ( 'NONE', #1403, .T. ) ;
#2914=DIRECTION ( 'NONE',  ( -0.000000000000000000, 1.000000000000000000, -0.000000000000000000 ) ) ;
#2916=CARTESIAN_POINT ( 'NONE',  ( 395.0000000000000000, -8.660254037844389075, 140.0000000000000000 ) ) ;
#2922=ORIENTED_EDGE ( 'NONE', *, *, #54, .F. ) ;
#2930=LINE ( 'NONE', #2515, #4812 ) ;
#2932=ORIENTED_EDGE ( 'NONE', *, *, #5619, .T. ) ;
#2935=DIRECTION ( 'NONE',  ( 0.000000000000000000, -1.000000000000000000, 0.000000000000000000 ) ) ;
#2936=DIRECTION ( 'NONE',  ( 0.000000000000000000, 0.000000000000000000, 1.000000000000000000 ) ) ;
#2939=CARTESIAN_POINT ( 'NONE',  ( 205.0000000000000284, 8.660254037844390851, 139.9990000000000236 ) ) ;
#2942=DIRECTION ( 'NONE',  ( -0.000000000000000000, 1.000000000000000000, 0.000000000000000000 ) ) ;
#2948=EDGE_LOOP ( 'NONE', ( #4141, #1374, #2232, #469 ) ) ;
#2951=VERTEX_POINT ( 'NONE', #4300 ) ;
#2953=ORIENTED_EDGE ( 'NONE', *, *, #4305, .T. ) ;
#2955=EDGE_CURVE ( 'NONE', #6476, #932, #5421, .T. ) ;
#2958=CARTESIAN_POINT ( 'NONE',  ( 285.0000000000000568, 8.660254037844390851, 139.9990000000000236 ) ) ;
#2960=LINE ( 'NONE', #1812, #532 ) ;
#2961=CARTESIAN_POINT ( 'NONE',  ( 164.9999999999999716, -8.660254037844389075, 140.0000000000000000 ) ) ;
#2964=DIRECTION ( 'NONE',  ( 0.000000000000000000, -1.000000000000000000, 0.000000000000000000 ) ) ;
#2965=LINE ( 'NONE', #5273, #1041 ) ;
#2972=EDGE_LOOP ( 'NONE', ( #4669, #4941, #237, #1332 ) ) ;
#2983=EDGE_LOOP ( 'NONE', ( #3146, #816, #3643, #6081 ) ) ;
#2987=ADVANCED_FACE ( 'NONE', ( #6039 ), #3281, .F. ) ;
#2990=VECTOR ( 'NONE', #2757, 1000.000000000000000 ) ;
#2991=EDGE_CURVE ( 'NONE', #3050, #1884, #467, .T. ) ;
#2992=ORIENTED_EDGE ( 'NONE', *, *, #4496, .F. ) ;
#2995=EDGE_CURVE ( 'NONE', #1933, #4178, #401, .T. ) ;
#2997=ORIENTED_EDGE ( 'NONE', *, *, #4389, .T. ) ;
#3005=CARTESIAN_POINT ( 'NONE',  ( -30.00000000000002842, -15.00000000000000000, 180.0000000000000284 ) ) ;
#3009=VECTOR ( 'NONE', #4037, 1000.000000000000000 ) ;
#3013=CARTESIAN_POINT ( 'NONE',  ( 405.0000000000000000, 8.660254037844390851, 139.9990000000000236 ) ) ;
#3014=FACE_OUTER_BOUND ( 'NONE', #4806, .T. ) ;
#3019=CARTESIAN_POINT ( 'NONE',  ( 53.33333333333330017, -14.99999999999999822, 165.1500000000000625 ) ) ;
#3023=VECTOR ( 'NONE', #873, 1000.000000000000000 ) ;
#3024=ORIENTED_EDGE ( 'NONE', *, *, #5965, .T. ) ;
#3030=AXIS2_PLACEMENT_3D ( 'NONE', #1211, #1181, #2845 ) ;
#3032=VERTEX_POINT ( 'NONE', #4479 ) ;
#3033=EDGE_CURVE ( 'NONE', #2062, #1523, #5043, .T. ) ;
#3036=DIRECTION ( 'NONE',  ( 0.000000000000000000, 1.000000000000000000, 0.000000000000000000 ) ) ;
#3038=DIRECTION ( 'NONE',  ( 0.000000000000000000, -1.000000000000000000, 0.000000000000000000 ) ) ;
#3044=CARTESIAN_POINT ( 'NONE',  ( -30.00000000000000000, 0.000000000000000000, 145.0000000000000284 ) ) ;
#3045=PLANE ( 'NONE',  #6008 ) ;
#3046=CARTESIAN_POINT ( 'NONE',  ( 285.0000000000000568, -8.660254037844389075, 139.9990000000000236 ) ) ;
#3050=VERTEX_POINT ( 'NONE', #2022 ) ;
#3051=ORIENTED_EDGE ( 'NONE', *, *, #6846, .F. ) ;
#3056=CARTESIAN_POINT ( 'NONE',  ( 219.9999999999999716, -20.00000000000000000, 165.1500000000000625 ) ) ;
#3059=VERTEX_POINT ( 'NONE', #6061 ) ;
#3062=ORIENTED_EDGE ( 'NONE', *, *, #3894, .T. ) ;
#3064=ORIENTED_EDGE ( 'NONE', *, *, #717, .T. ) ;
#3071=DIRECTION ( 'NONE',  ( -0.000000000000000000, -0.000000000000000000, 1.000000000000000000 ) ) ;
#3077=DIRECTION ( 'NONE',  ( 0.000000000000000000, -0.000000000000000000, -1.000000000000000000 ) ) ;
#3078=FACE_BOUND ( 'NONE', #5318, .T. ) ;
#3080=ORIENTED_EDGE ( 'NONE', *, *, #5380, .F. ) ;
#3082=ADVANCED_FACE ( 'NONE', ( #2180 ), #6096, .F. ) ;
#3085=DIRECTION ( 'NONE',  ( 1.000000000000000000, 0.000000000000000000, 0.000000000000000000 ) ) ;
#3086=PLANE ( 'NONE',  #2833 ) ;
#3091=ADVANCED_FACE ( 'NONE', ( #485 ), #3303, .F. ) ;
#3092=ORIENTED_EDGE ( 'NONE', *, *, #6, .F. ) ;
#3093=VECTOR ( 'NONE', #295, 1000.000000000000000 ) ;
#3100=FACE_OUTER_BOUND ( 'NONE', #1907, .T. ) ;
#3108=DIRECTION ( 'NONE',  ( -1.000000000000000000, 0.000000000000000000, 0.000000000000000000 ) ) ;
#3117=CARTESIAN_POINT ( 'NONE',  ( 435.0000000000000568, -8.660254037844389075, 139.9990000000000236 ) ) ;
#3118=DIRECTION ( 'NONE',  ( 1.000000000000000000, 0.000000000000000000, 0.000000000000000000 ) ) ;
#3127=CARTESIAN_POINT ( 'NONE',  ( 325.0000000000000000, 8.660254037844390851, 140.0000000000000000 ) ) ;
#3135=CARTESIAN_POINT ( 'NONE',  ( 405.0000000000000000, 8.660254037844390851, 145.0000000000000284 ) ) ;
#3136=ADVANCED_FACE ( 'NONE', ( #4655 ), #4365, .F. ) ;
#3138=VECTOR ( 'NONE', #6201, 1000.000000000000000 ) ;
#3139=CARTESIAN_POINT ( 'NONE',  ( -5.000000000000000888, -8.660254037844389075, 145.0000000000000284 ) ) ;
#3141=EDGE_CURVE ( 'NONE', #3817, #2951, #6845, .T. ) ;
#3142=LINE ( 'NONE', #4970, #4246 ) ;
#3146=ORIENTED_EDGE ( 'NONE', *, *, #4343, .F. ) ;
#3153=CARTESIAN_POINT ( 'NONE',  ( 75.00000000000001421, 8.660254037844390851, 145.0000000000000284 ) ) ;
#3156=PLANE ( 'NONE',  #6399 ) ;
#3158=VERTEX_POINT ( 'NONE', #6884 ) ;
#3159=LINE ( 'NONE', #825, #4092 ) ;
#3160=ORIENTED_EDGE ( 'NONE', *, *, #1783, .T. ) ;
#3170=ORIENTED_EDGE ( 'NONE', *, *, #5009, .F. ) ;
#3172=DIRECTION ( 'NONE',  ( -1.000000000000000000, -0.000000000000000000, -0.000000000000000000 ) ) ;
#3173=ORIENTED_EDGE ( 'NONE', *, *, #5313, .F. ) ;
#3174=DIRECTION ( 'NONE',  ( -0.000000000000000000, 1.000000000000000000, -0.000000000000000000 ) ) ;
#3175=( NAMED_UNIT ( * ) SI_UNIT ( $, .STERADIAN. ) SOLID_ANGLE_UNIT ( ) );
#3176=CARTESIAN_POINT ( 'NONE',  ( 195.0000000000000000, 8.660254037844390851, 139.9990000000000236 ) ) ;
#3179=EDGE_LOOP ( 'NONE', ( #3199, #5535, #527, #5223 ) ) ;
#3181=ORIENTED_EDGE ( 'NONE', *, *, #6862, .F. ) ;
#3183=LINE ( 'NONE', #335, #1618 ) ;
#3184=DIRECTION ( 'NONE',  ( 0.000000000000000000, 0.000000000000000000, 1.000000000000000000 ) ) ;
#3186=EDGE_CURVE ( 'NONE', #6064, #1325, #5637, .T. ) ;
#3189=MANIFOLD_SOLID_BREP ( 'M5 Clearance Hole1', #3615 ) ;
#3192=CARTESIAN_POINT ( 'NONE',  ( 4.999999999999999112, -8.660254037844389075, 139.9990000000000236 ) ) ;
#3199=ORIENTED_EDGE ( 'NONE', *, *, #7244, .T. ) ;
#3203=DIRECTION ( 'NONE',  ( 1.000000000000000000, 0.000000000000000000, 0.000000000000000000 ) ) ;
#3205=CARTESIAN_POINT ( 'NONE',  ( 75.00000000000001421, 8.660254037844390851, 139.9990000000000236 ) ) ;
#3206=VERTEX_POINT ( 'NONE', #1216 ) ;
#3207=CARTESIAN_POINT ( 'NONE',  ( 355.0000000000000000, 8.660254037844390851, 139.9990000000000236 ) ) ;
#3208=DIRECTION ( 'NONE',  ( -0.000000000000000000, 1.000000000000000000, -0.000000000000000000 ) ) ;
#3214=AXIS2_PLACEMENT_3D ( 'NONE', #5632, #2478, #3646 ) ;
#3215=AXIS2_PLACEMENT_3D ( 'NONE', #225, #1267, #4145 ) ;
#3216=ORIENTED_EDGE ( 'NONE', *, *, #6455, .T. ) ;
#3220=LINE ( 'NONE', #5981, #4724 ) ;
#3223=EDGE_CURVE ( 'NONE', #732, #7234, #2327, .T. ) ;
#3231=FACE_BOUND ( 'NONE', #3433, .T. ) ;
#3235=DIRECTION ( 'NONE',  ( 1.000000000000000000, 0.000000000000000000, 0.000000000000000000 ) ) ;
#3236=VECTOR ( 'NONE', #4869, 1000.000000000000000 ) ;
#3237=ORIENTED_EDGE ( 'NONE', *, *, #1373, .F. ) ;
#3245=DIRECTION ( 'NONE',  ( -0.000000000000000000, 1.000000000000000000, -0.000000000000000000 ) ) ;
#3246=PLANE ( 'NONE',  #1353 ) ;
#3248=EDGE_CURVE ( 'NONE', #6476, #1413, #1354, .T. ) ;
#3249=CARTESIAN_POINT ( 'NONE',  ( 355.0000000000000000, 8.660254037844390851, 139.9990000000000236 ) ) ;
#3250=VECTOR ( 'NONE', #3549, 1000.000000000000000 ) ;
#3253=CIRCLE ( 'NONE', #539, 2.649999999999985700 ) ;
#3254=FACE_OUTER_BOUND ( 'NONE', #406, .T. ) ;
#3256=VECTOR ( 'NONE', #5592, 1000.000000000000000 ) ;
#3260=ORIENTED_EDGE ( 'NONE', *, *, #5695, .F. ) ;
#3261=VERTEX_POINT ( 'NONE', #5327 ) ;
#3263=ORIENTED_EDGE ( 'NONE', *, *, #7216, .T. ) ;
#3265=MECHANICAL_DESIGN_GEOMETRIC_PRESENTATION_REPRESENTATION('',(#547),#2316);
#3266=CARTESIAN_POINT ( 'NONE',  ( 386.6666666666666288, -14.99999999999999822, 165.1500000000000625 ) ) ;
#3268=DIRECTION ( 'NONE',  ( 1.000000000000000000, 0.000000000000000000, 0.000000000000000000 ) ) ;
#3269=ADVANCED_FACE ( 'NONE', ( #4764 ), #6384, .F. ) ;
#3270=SHAPE_REPRESENTATION ( 'side rail', ( #1963 ), #5422 ) ;
#3272=EDGE_LOOP ( 'NONE', ( #5025, #3260, #6298, #591 ) ) ;
#3275=PLANE ( 'NONE',  #4327 ) ;
#3276=CARTESIAN_POINT ( 'NONE',  ( 275.0000000000000000, -8.660254037844389075, 145.0000000000000284 ) ) ;
#3281=PLANE ( 'NONE',  #5408 ) ;
#3285=ORIENTED_EDGE ( 'NONE', *, *, #3141, .F. ) ;
#3286=FACE_OUTER_BOUND ( 'NONE', #1237, .T. ) ;
#3288=PLANE ( 'NONE',  #1506 ) ;
#3289=CARTESIAN_POINT ( 'NONE',  ( 75.00000000000001421, 8.660254037844390851, 139.9990000000000236 ) ) ;
#3290=DIRECTION ( 'NONE',  ( -1.000000000000000000, 0.000000000000000000, 0.000000000000000000 ) ) ;
#3293=CARTESIAN_POINT ( 'NONE',  ( -5.000000000000000888, 8.660254037844390851, 140.0000000000000000 ) ) ;
#3294=VECTOR ( 'NONE', #6670, 1000.000000000000000 ) ;
#3300=CARTESIAN_POINT ( 'NONE',  ( 365.0000000000000000, 8.660254037844390851, 140.0000000000000000 ) ) ;
#3303=PLANE ( 'NONE',  #1343 ) ;
#3309=VERTEX_POINT ( 'NONE', #3667 ) ;
#3311=FACE_OUTER_BOUND ( 'NONE', #270, .T. ) ;
#3312=CARTESIAN_POINT ( 'NONE',  ( 303.3333333333333144, -14.99999999999999822, 159.8500000000001080 ) ) ;
#3313=ORIENTED_EDGE ( 'NONE', *, *, #2907, .T. ) ;
#3315=SHAPE_DEFINITION_REPRESENTATION ( #1929, #3270 ) ;
#3318=LINE ( 'NONE', #9, #1957 ) ;
#3337=DIRECTION ( 'NONE',  ( 0.000000000000000000, 0.000000000000000000, 1.000000000000000000 ) ) ;
#3339=DIRECTION ( 'NONE',  ( 1.000000000000000000, 0.000000000000000000, 0.000000000000000000 ) ) ;
#3340=ORIENTED_EDGE ( 'NONE', *, *, #5545, .T. ) ;
#3341=EDGE_CURVE ( 'NONE', #4268, #1111, #5360, .T. ) ;
#3343=VECTOR ( 'NONE', #2804, 1000.000000000000000 ) ;
#3345=EDGE_LOOP ( 'NONE', ( #736, #1077, #6071, #3173 ) ) ;
#3348=CARTESIAN_POINT ( 'NONE',  ( 205.0000000000000284, 8.660254037844390851, 139.9990000000000236 ) ) ;
#3356=DIRECTION ( 'NONE',  ( 0.000000000000000000, -1.000000000000000000, 0.000000000000000000 ) ) ;
#3357=ADVANCED_FACE ( 'NONE', ( #4833 ), #6456, .F. ) ;
#3367=AXIS2_PLACEMENT_3D ( 'NONE', #1817, #2482, #6337 ) ;
#3368=ADVANCED_FACE ( 'NONE', ( #1394 ), #5287, .F. ) ;
#3372=LINE ( 'NONE', #444, #3766 ) ;
#3374=CARTESIAN_POINT ( 'NONE',  ( 386.6666666666666288, -15.00000000000000000, 162.5000000000000853 ) ) ;
#3377=VERTEX_POINT ( 'NONE', #3019 ) ;
#3378=STYLED_ITEM('',(#7425),#3189);
#3380=ORIENTED_EDGE ( 'NONE', *, *, #3560, .F. ) ;
#3386=VERTEX_POINT ( 'NONE', #6817 ) ;
#3397=VERTEX_POINT ( 'NONE', #4686 ) ;
#3401=EDGE_CURVE ( 'NONE', #4768, #1782, #6424, .T. ) ;
#3403=CARTESIAN_POINT ( 'NONE',  ( 275.0000000000000000, 8.660254037844390851, 145.0000000000000284 ) ) ;
#3404=DIRECTION ( 'NONE',  ( -0.000000000000000000, 0.000000000000000000, 1.000000000000000000 ) ) ;
#3405=VECTOR ( 'NONE', #1165, 1000.000000000000000 ) ;
#3407=DIRECTION ( 'NONE',  ( 1.000000000000000000, 0.000000000000000000, 0.000000000000000000 ) ) ;
#3409=ORIENTED_EDGE ( 'NONE', *, *, #4152, .T. ) ;
#3410=CARTESIAN_POINT ( 'NONE',  ( 195.0000000000000000, -8.660254037844389075, 139.9990000000000236 ) ) ;
#3411=EDGE_LOOP ( 'NONE', ( #704, #5064, #1024, #1991 ) ) ;
#3412=VECTOR ( 'NONE', #1203, 1000.000000000000000 ) ;
#3414=FACE_BOUND ( 'NONE', #6937, .T. ) ;
#3416=DIRECTION ( 'NONE',  ( 0.000000000000000000, 0.000000000000000000, 1.000000000000000000 ) ) ;
#3418=EDGE_CURVE ( 'NONE', #1782, #5777, #4730, .T. ) ;
#3419=VECTOR ( 'NONE', #2753, 1000.000000000000000 ) ;
#3421=ORIENTED_EDGE ( 'NONE', *, *, #7080, .F. ) ;
#3423=VECTOR ( 'NONE', #4367, 1000.000000000000000 ) ;
#3425=LINE ( 'NONE', #2119, #1260 ) ;
#3427=CARTESIAN_POINT ( 'NONE',  ( 245.0000000000000000, -8.660254037844389075, 140.0000000000000000 ) ) ;
#3428=VERTEX_POINT ( 'NONE', #6452 ) ;
#3429=LINE ( 'NONE', #529, #2990 ) ;
#3430=LINE ( 'NONE', #6752, #305 ) ;
#3432=EDGE_CURVE ( 'NONE', #266, #4461, #274, .T. ) ;
#3433=EDGE_LOOP ( 'NONE', ( #6863, #95, #2831, #1990 ) ) ;
#3440=CARTESIAN_POINT ( 'NONE',  ( 245.0000000000000000, 8.660254037844390851, 139.9990000000000236 ) ) ;
#3442=ORIENTED_EDGE ( 'NONE', *, *, #4112, .T. ) ;
#3445=FACE_BOUND ( 'NONE', #2476, .T. ) ;
#3446=DIRECTION ( 'NONE',  ( 0.000000000000000000, 0.000000000000000000, 1.000000000000000000 ) ) ;
#3450=ORIENTED_EDGE ( 'NONE', *, *, #13, .F. ) ;
#3453=ORIENTED_EDGE ( 'NONE', *, *, #6923, .T. ) ;
#3455=DIRECTION ( 'NONE',  ( -0.000000000000000000, -0.000000000000000000, 1.000000000000000000 ) ) ;
#3460=CARTESIAN_POINT ( 'NONE',  ( 84.99999999999998579, 8.660254037844390851, 139.9990000000000236 ) ) ;
#3461=VERTEX_POINT ( 'NONE', #5968 ) ;
#3466=VERTEX_POINT ( 'NONE', #5887 ) ;
#3468=LINE ( 'NONE', #194, #155 ) ;
#3469=DIRECTION ( 'NONE',  ( 0.000000000000000000, 0.000000000000000000, 1.000000000000000000 ) ) ;
#3470=CARTESIAN_POINT ( 'NONE',  ( 75.00000000000001421, 8.660254037844390851, 140.0000000000000000 ) ) ;
#3472=ORIENTED_EDGE ( 'NONE', *, *, #2272, .T. ) ;
#3475=ORIENTED_EDGE ( 'NONE', *, *, #6441, .F. ) ;
#3480=VECTOR ( 'NONE', #4645, 1000.000000000000000 ) ;
#3486=LINE ( 'NONE', #2361, #1939 ) ;
#3487=ORIENTED_EDGE ( 'NONE', *, *, #368, .T. ) ;
#3489=LINE ( 'NONE', #3563, #573 ) ;
#3503=LINE ( 'NONE', #50, #4981 ) ;
#3505=DIRECTION ( 'NONE',  ( -0.000000000000000000, 1.000000000000000000, -0.000000000000000000 ) ) ;
#3506=LINE ( 'NONE', #3046, #3634 ) ;
#3507=VECTOR ( 'NONE', #5491, 1000.000000000000000 ) ;
#3509=VERTEX_POINT ( 'NONE', #2464 ) ;
#3512=ORIENTED_EDGE ( 'NONE', *, *, #3186, .F. ) ;
#3516=CARTESIAN_POINT ( 'NONE',  ( 386.6666666666666288, -20.00000000000000000, 162.5000000000000853 ) ) ;
#3519=AXIS2_PLACEMENT_3D ( 'NONE', #4, #1564, #1639 ) ;
#3524=CARTESIAN_POINT ( 'NONE',  ( 445.0000000000000000, 8.660254037844390851, 139.9990000000000236 ) ) ;
#3536=EDGE_CURVE ( 'NONE', #1502, #7340, #5357, .T. ) ;
#3540=LINE ( 'NONE', #5919, #2879 ) ;
#3541=CARTESIAN_POINT ( 'NONE',  ( -30.00000000000002842, -15.00000000000000000, 145.0000000000000284 ) ) ;
#3542=ORIENTED_EDGE ( 'NONE', *, *, #24, .T. ) ;
#3543=CARTESIAN_POINT ( 'NONE',  ( 136.6666666666666288, -14.99999999999999822, 162.5000000000000853 ) ) ;
#3547=CARTESIAN_POINT ( 'NONE',  ( 155.0000000000000000, 8.660254037844390851, 139.9990000000000236 ) ) ;
#3549=DIRECTION ( 'NONE',  ( 0.000000000000000000, 1.000000000000000000, 0.000000000000000000 ) ) ;
#3553=EDGE_CURVE ( 'NONE', #2018, #1972, #4908, .T. ) ;
#3555=ORIENTED_EDGE ( 'NONE', *, *, #2701, .F. ) ;
#3558=CARTESIAN_POINT ( 'NONE',  ( -30.00000000000002842, 15.00000000000000000, 140.0000000000000000 ) ) ;
#3559=ORIENTED_EDGE ( 'NONE', *, *, #4340, .F. ) ;
#3560=EDGE_CURVE ( 'NONE', #4557, #5461, #1030, .T. ) ;
#3563=CARTESIAN_POINT ( 'NONE',  ( 84.99999999999998579, -8.660254037844389075, 139.9990000000000236 ) ) ;
#3565=DIRECTION ( 'NONE',  ( 0.000000000000000000, 0.000000000000000000, -1.000000000000000000 ) ) ;
#3587=LINE ( 'NONE', #5248, #427 ) ;
#3588=DIRECTION ( 'NONE',  ( 0.000000000000000000, -0.000000000000000000, 1.000000000000000000 ) ) ;
#3589=EDGE_CURVE ( 'NONE', #5499, #4862, #7196, .T. ) ;
#3593=EDGE_LOOP ( 'NONE', ( #4725, #5527, #2596, #925 ) ) ;
#3607=ORIENTED_EDGE ( 'NONE', *, *, #7038, .F. ) ;
#3608=CARTESIAN_POINT ( 'NONE',  ( 114.9999999999999858, -8.660254037844389075, 140.0000000000000000 ) ) ;
#3615=CLOSED_SHELL ( 'NONE', ( #915, #788, #2085, #1558, #5890, #1733, #2237, #244, #3987, #3798, #4726, #3368, #5130, #4033, #6274, #4489, #6732, #5730, #2130, #7232, #4170, #1626, #4374, #4889, #1941, #3269, #6428, #5261, #1899, #3678, #2750, #3091, #7263, #4781, #6289, #1287, #2192, #5343, #6631, #3082, #1779, #3136, #7093, #2549, #3924, #4959, #2584, #3901, #5918, #6713, #4045, #4635, #1404, #1988, #4702, #2987, #4661, #223, #826, #1107, #1191, #6478, #4293, #3357, #4473, #276 ) ) ;
#3622=CARTESIAN_POINT ( 'NONE',  ( 355.0000000000000000, 8.660254037844390851, 145.0000000000000284 ) ) ;
#3625=EDGE_LOOP ( 'NONE', ( #325, #595, #4094, #5341 ) ) ;
#3626=LINE ( 'NONE', #165, #1323 ) ;
#3634=VECTOR ( 'NONE', #1274, 1000.000000000000000 ) ;
#3636=ORIENTED_EDGE ( 'NONE', *, *, #6184, .T. ) ;
#3639=EDGE_CURVE ( 'NONE', #6561, #1168, #6718, .T. ) ;
#3642=PLANE ( 'NONE',  #782 ) ;
#3643=ORIENTED_EDGE ( 'NONE', *, *, #193, .T. ) ;
#3644=VECTOR ( 'NONE', #2765, 1000.000000000000000 ) ;
#3646=DIRECTION ( 'NONE',  ( -0.000000000000000000, 0.000000000000000000, 1.000000000000000000 ) ) ;
#3647=DIRECTION ( 'NONE',  ( 0.000000000000000000, -0.000000000000000000, 1.000000000000000000 ) ) ;
#3654=EDGE_LOOP ( 'NONE', ( #1227, #236, #1822, #2849 ) ) ;
#3655=LINE ( 'NONE', #5454, #6981 ) ;
#3657=DIRECTION ( 'NONE',  ( -0.000000000000000000, 1.000000000000000000, -0.000000000000000000 ) ) ;
#3658=EDGE_CURVE ( 'NONE', #5826, #7027, #985, .T. ) ;
#3659=ORIENTED_EDGE ( 'NONE', *, *, #2403, .T. ) ;
#3660=DIRECTION ( 'NONE',  ( 1.000000000000000000, 0.000000000000000000, 0.000000000000000000 ) ) ;
#3662=EDGE_LOOP ( 'NONE', ( #2380, #6117, #900, #3285 ) ) ;
#3663=FACE_OUTER_BOUND ( 'NONE', #5937, .T. ) ;
#3667=CARTESIAN_POINT ( 'NONE',  ( -30.00000000000002842, -20.00000000000000000, 180.0000000000000284 ) ) ;
#3668=DIRECTION ( 'NONE',  ( -0.000000000000000000, -0.000000000000000000, 1.000000000000000000 ) ) ;
#3669=EDGE_LOOP ( 'NONE', ( #3475, #1874, #5685, #2922 ) ) ;
#3673=VERTEX_POINT ( 'NONE', #7158 ) ;
#3675=FILL_AREA_STYLE_COLOUR ( '', #662 ) ;
#3678=ADVANCED_FACE ( 'NONE', ( #2168 ), #472, .F. ) ;
#3679=ORIENTED_EDGE ( 'NONE', *, *, #2225, .F. ) ;
#3681=DIRECTION ( 'NONE',  ( -1.000000000000000000, -0.000000000000000000, -0.000000000000000000 ) ) ;
#3684=LINE ( 'NONE', #2121, #6539 ) ;
#3685=EDGE_LOOP ( 'NONE', ( #2588, #1095, #5352, #5986 ) ) ;
#3689=CARTESIAN_POINT ( 'NONE',  ( 355.0000000000000000, -8.660254037844389075, 139.9990000000000236 ) ) ;
#3690=FACE_BOUND ( 'NONE', #4982, .T. ) ;
#3697=VERTEX_POINT ( 'NONE', #5660 ) ;
#3701=FACE_OUTER_BOUND ( 'NONE', #811, .T. ) ;
#3702=EDGE_CURVE ( 'NONE', #4019, #6406, #5770, .T. ) ;
#3714=EDGE_LOOP ( 'NONE', ( #5212, #3062, #4302, #4109 ) ) ;
#3722=VERTEX_POINT ( 'NONE', #5111 ) ;
#3737=PLANE ( 'NONE',  #5628 ) ;
#3738=PLANE ( 'NONE',  #1262 ) ;
#3739=DIRECTION ( 'NONE',  ( -0.000000000000000000, -0.000000000000000000, 1.000000000000000000 ) ) ;
#3743=AXIS2_PLACEMENT_3D ( 'NONE', #6105, #6624, #3184 ) ;
#3745=CARTESIAN_POINT ( 'NONE',  ( -5.000000000000000888, 8.660254037844390851, 145.0000000000000284 ) ) ;
#3751=VECTOR ( 'NONE', #6531, 1000.000000000000000 ) ;
#3754=CARTESIAN_POINT ( 'NONE',  ( 114.9999999999999858, 8.660254037844390851, 139.9990000000000236 ) ) ;
#3764=VECTOR ( 'NONE', #6927, 1000.000000000000000 ) ;
#3765=ORIENTED_EDGE ( 'NONE', *, *, #1567, .T. ) ;
#3766=VECTOR ( 'NONE', #1552, 1000.000000000000000 ) ;
#3768=DIRECTION ( 'NONE',  ( -0.000000000000000000, 0.000000000000000000, 1.000000000000000000 ) ) ;
#3770=ORIENTED_EDGE ( 'NONE', *, *, #1768, .F. ) ;
#3773=CARTESIAN_POINT ( 'NONE',  ( 355.0000000000000000, 8.660254037844390851, 139.9990000000000236 ) ) ;
#3778=EDGE_CURVE ( 'NONE', #4228, #6725, #2245, .T. ) ;
#3779=EDGE_LOOP ( 'NONE', ( #2745, #7138 ) ) ;
#3783=DIRECTION ( 'NONE',  ( 1.000000000000000000, 0.000000000000000000, 0.000000000000000000 ) ) ;
#3789=ORIENTED_EDGE ( 'NONE', *, *, #2003, .F. ) ;
#3792=LINE ( 'NONE', #806, #3875 ) ;
#3796=DIRECTION ( 'NONE',  ( -0.000000000000000000, 1.000000000000000000, 0.000000000000000000 ) ) ;
#3798=ADVANCED_FACE ( 'NONE', ( #1705 ), #524, .F. ) ;
#3799=ORIENTED_EDGE ( 'NONE', *, *, #4602, .F. ) ;
#3810=PLANE ( 'NONE',  #6960 ) ;
#3811=FACE_OUTER_BOUND ( 'NONE', #1568, .T. ) ;
#3815=EDGE_CURVE ( 'NONE', #732, #4657, #1619, .T. ) ;
#3817=VERTEX_POINT ( 'NONE', #6907 ) ;
#3826=VERTEX_POINT ( 'NONE', #4574 ) ;
#3827=DIRECTION ( 'NONE',  ( -0.000000000000000000, 1.000000000000000000, -0.000000000000000000 ) ) ;
#3829=DIRECTION ( 'NONE',  ( -0.000000000000000000, -0.000000000000000000, 1.000000000000000000 ) ) ;
#3836=AXIS2_PLACEMENT_3D ( 'NONE', #28, #222, #2252 ) ;
#3842=CARTESIAN_POINT ( 'NONE',  ( -30.00000000000002842, -15.00000000000000000, 140.0000000000000000 ) ) ;
#3843=EDGE_CURVE ( 'NONE', #4557, #4971, #2312, .T. ) ;
#3853=EDGE_CURVE ( 'NONE', #5777, #1731, #5206, .T. ) ;
#3856=VECTOR ( 'NONE', #2210, 1000.000000000000000 ) ;
#3858=ORIENTED_EDGE ( 'NONE', *, *, #6230, .F. ) ;
#3860=CARTESIAN_POINT ( 'NONE',  ( 195.0000000000000000, 8.660254037844390851, 140.0000000000000000 ) ) ;
#3862=DIRECTION ( 'NONE',  ( 1.000000000000000000, 0.000000000000000000, 0.000000000000000000 ) ) ;
#3863=CARTESIAN_POINT ( 'NONE',  ( 315.0000000000000568, 8.660254037844390851, 145.0000000000000284 ) ) ;
#3865=VECTOR ( 'NONE', #3339, 1000.000000000000000 ) ;
#3867=DIRECTION ( 'NONE',  ( -1.000000000000000000, -0.000000000000000000, 0.000000000000000000 ) ) ;
#3868=VECTOR ( 'NONE', #3038, 1000.000000000000000 ) ;
#3869=VERTEX_POINT ( 'NONE', #1787 ) ;
#3870=DIRECTION ( 'NONE',  ( -0.000000000000000000, -0.000000000000000000, 1.000000000000000000 ) ) ;
#3871=DIRECTION ( 'NONE',  ( -0.000000000000000000, 1.000000000000000000, -0.000000000000000000 ) ) ;
#3875=VECTOR ( 'NONE', #3172, 1000.000000000000000 ) ;
#3878=VECTOR ( 'NONE', #7020, 1000.000000000000000 ) ;
#3879=ORIENTED_EDGE ( 'NONE', *, *, #6230, .T. ) ;
#3885=CARTESIAN_POINT ( 'NONE',  ( 395.0000000000000000, 8.660254037844390851, 145.0000000000000284 ) ) ;
#3886=DIRECTION ( 'NONE',  ( -0.000000000000000000, 1.000000000000000000, 0.000000000000000000 ) ) ;
#3887=CARTESIAN_POINT ( 'NONE',  ( 114.9999999999999858, -8.660254037844389075, 145.0000000000000284 ) ) ;
#3888=VECTOR ( 'NONE', #4777, 1000.000000000000000 ) ;
#3894=EDGE_CURVE ( 'NONE', #183, #3673, #3540, .T. ) ;
#3901=ADVANCED_FACE ( 'NONE', ( #2414 ), #684, .F. ) ;
#3906=DIRECTION ( 'NONE',  ( -0.000000000000000000, -0.000000000000000000, 1.000000000000000000 ) ) ;
#3908=CARTESIAN_POINT ( 'NONE',  ( -5.000000000000000888, 8.660254037844390851, 139.9990000000000236 ) ) ;
#3910=DIRECTION ( 'NONE',  ( -0.000000000000000000, -0.000000000000000000, 1.000000000000000000 ) ) ;
#3916=FACE_BOUND ( 'NONE', #3669, .T. ) ;
#3920=VERTEX_POINT ( 'NONE', #229 ) ;
#3922=ORIENTED_EDGE ( 'NONE', *, *, #96, .T. ) ;
#3924=ADVANCED_FACE ( 'NONE', ( #263 ), #3045, .F. ) ;
#3925=DIRECTION ( 'NONE',  ( 0.000000000000000000, 1.000000000000000000, 0.000000000000000000 ) ) ;
#3929=CYLINDRICAL_SURFACE ( 'NONE', #314, 2.649999999999985700 ) ;
#3937=ORIENTED_EDGE ( 'NONE', *, *, #1248, .F. ) ;
#3943=DIRECTION ( 'NONE',  ( -0.000000000000000000, 1.000000000000000000, -0.000000000000000000 ) ) ;
#3947=ORIENTED_EDGE ( 'NONE', *, *, #1567, .F. ) ;
#3949=EDGE_CURVE ( 'NONE', #6959, #2007, #6965, .T. ) ;
#3951=DIRECTION ( 'NONE',  ( 0.000000000000000000, 0.000000000000000000, 1.000000000000000000 ) ) ;
#3956=EDGE_LOOP ( 'NONE', ( #6020, #3799, #6175, #6217, #5641, #2582 ) ) ;
#3964=PLANE ( 'NONE',  #4626 ) ;
#3969=CARTESIAN_POINT ( 'NONE',  ( -5.000000000000000888, 8.660254037844390851, 145.0000000000000284 ) ) ;
#3971=ORIENTED_EDGE ( 'NONE', *, *, #2721, .T. ) ;
#3972=CARTESIAN_POINT ( 'NONE',  ( 235.0000000000000000, 8.660254037844390851, 140.0000000000000000 ) ) ;
#3973=EDGE_CURVE ( 'NONE', #4758, #6476, #2125, .T. ) ;
#3976=DIRECTION ( 'NONE',  ( 0.000000000000000000, 1.000000000000000000, 0.000000000000000000 ) ) ;
#3978=CARTESIAN_POINT ( 'NONE',  ( 35.00000000000000000, 8.660254037844390851, 145.0000000000000284 ) ) ;
#3980=ORIENTED_EDGE ( 'NONE', *, *, #4529, .T. ) ;
#3982=VERTEX_POINT ( 'NONE', #1448 ) ;
#3987=ADVANCED_FACE ( 'NONE', ( #5578 ), #3810, .F. ) ;
#3991=ORIENTED_EDGE ( 'NONE', *, *, #54, .T. ) ;
#4002=AXIS2_PLACEMENT_3D ( 'NONE', #3374, #2220, #3337 ) ;
#4011=VERTEX_POINT ( 'NONE', #1534 ) ;
#4014=VECTOR ( 'NONE', #4455, 1000.000000000000000 ) ;
#4017=FACE_OUTER_BOUND ( 'NONE', #1434, .T. ) ;
#4019=VERTEX_POINT ( 'NONE', #7112 ) ;
#4021=EDGE_CURVE ( 'NONE', #2157, #6398, #4895, .T. ) ;
#4024=CARTESIAN_POINT ( 'NONE',  ( 365.0000000000000000, 8.660254037844390851, 139.9990000000000236 ) ) ;
#4027=VECTOR ( 'NONE', #771, 1000.000000000000000 ) ;
#4031=ORIENTED_EDGE ( 'NONE', *, *, #5545, .F. ) ;
#4033=ADVANCED_FACE ( 'NONE', ( #5455 ), #1495, .F. ) ;
#4037=DIRECTION ( 'NONE',  ( 0.000000000000000000, -1.000000000000000000, 0.000000000000000000 ) ) ;
#4041=LINE ( 'NONE', #683, #913 ) ;
#4045=ADVANCED_FACE ( 'NONE', ( #2684 ), #3275, .T. ) ;
#4046=ORIENTED_EDGE ( 'NONE', *, *, #2728, .T. ) ;
#4048=VERTEX_POINT ( 'NONE', #5990 ) ;
#4049=PLANE ( 'NONE',  #382 ) ;
#4051=LINE ( 'NONE', #6239, #373 ) ;
#4057=EDGE_LOOP ( 'NONE', ( #5438, #2658, #5224, #4991 ) ) ;
#4059=EDGE_CURVE ( 'NONE', #7144, #4178, #4380, .T. ) ;
#4064=LINE ( 'NONE', #1778, #2208 ) ;
#4066=EDGE_LOOP ( 'NONE', ( #2932, #6715, #5046, #3559 ) ) ;
#4068=DIRECTION ( 'NONE',  ( 1.000000000000000000, 0.000000000000000000, 0.000000000000000000 ) ) ;
#4071=AXIS2_PLACEMENT_3D ( 'NONE', #5595, #3827, #1469 ) ;
#4073=DIRECTION ( 'NONE',  ( 0.000000000000000000, -0.000000000000000000, -1.000000000000000000 ) ) ;
#4080=DIRECTION ( 'NONE',  ( -0.000000000000000000, 1.000000000000000000, -0.000000000000000000 ) ) ;
#4081=EDGE_LOOP ( 'NONE', ( #6931, #3555, #2291, #2834 ) ) ;
#4083=CARTESIAN_POINT ( 'NONE',  ( 275.0000000000000000, -8.660254037844389075, 140.0000000000000000 ) ) ;
#4085=LINE ( 'NONE', #4549, #2501 ) ;
#4087=VECTOR ( 'NONE', #3906, 1000.000000000000000 ) ;
#4089=EDGE_LOOP ( 'NONE', ( #2953, #3024, #1025, #6359 ) ) ;
#4092=VECTOR ( 'NONE', #3235, 1000.000000000000000 ) ;
#4094=ORIENTED_EDGE ( 'NONE', *, *, #96, .F. ) ;
#4096=VECTOR ( 'NONE', #516, 1000.000000000000000 ) ;
#4098=DIRECTION ( 'NONE',  ( 0.000000000000000000, -1.000000000000000000, 0.000000000000000000 ) ) ;
#4105=VECTOR ( 'NONE', #4787, 1000.000000000000000 ) ;
#4106=LINE ( 'NONE', #6437, #3868 ) ;
#4109=ORIENTED_EDGE ( 'NONE', *, *, #3418, .F. ) ;
#4112=EDGE_CURVE ( 'NONE', #3509, #6334, #812, .T. ) ;
#4115=CARTESIAN_POINT ( 'NONE',  ( 0.000000000000000000, 15.00000000000000000, 145.0000000000000284 ) ) ;
#4116=DIRECTION ( 'NONE',  ( -0.000000000000000000, 1.000000000000000000, 0.000000000000000000 ) ) ;
#4117=VECTOR ( 'NONE', #2485, 1000.000000000000000 ) ;
#4124=VECTOR ( 'NONE', #7305, 1000.000000000000000 ) ;
#4126=DIRECTION ( 'NONE',  ( -0.000000000000000000, -0.000000000000000000, 1.000000000000000000 ) ) ;
#4128=CARTESIAN_POINT ( 'NONE',  ( 285.0000000000000568, 8.660254037844390851, 140.0000000000000000 ) ) ;
#4131=DIRECTION ( 'NONE',  ( -0.000000000000000000, -0.000000000000000000, 1.000000000000000000 ) ) ;
#4132=VECTOR ( 'NONE', #6170, 1000.000000000000000 ) ;
#4133=EDGE_LOOP ( 'NONE', ( #343, #1742, #2204, #466 ) ) ;
#4136=ORIENTED_EDGE ( 'NONE', *, *, #2234, .T. ) ;
#4137=VECTOR ( 'NONE', #3783, 1000.000000000000000 ) ;
#4141=ORIENTED_EDGE ( 'NONE', *, *, #1248, .T. ) ;
#4143=CARTESIAN_POINT ( 'NONE',  ( 386.6666666666666288, -15.00000000000000000, 159.8500000000001080 ) ) ;
#4145=DIRECTION ( 'NONE',  ( 0.000000000000000000, 0.000000000000000000, 1.000000000000000000 ) ) ;
#4150=CARTESIAN_POINT ( 'NONE',  ( 75.00000000000001421, 8.660254037844390851, 139.9990000000000236 ) ) ;
#4152=EDGE_CURVE ( 'NONE', #1397, #6725, #5948, .T. ) ;
#4153=ORIENTED_EDGE ( 'NONE', *, *, #6741, .F. ) ;
#4155=PRODUCT ( 'side rail', 'side rail', '', ( #5225 ) ) ;
#4158=ORIENTED_EDGE ( 'NONE', *, *, #6699, .F. ) ;
#4159=LINE ( 'NONE', #6938, #4915 ) ;
#4164=DIRECTION ( 'NONE',  ( 0.000000000000000000, -1.000000000000000000, 0.000000000000000000 ) ) ;
#4166=EDGE_LOOP ( 'NONE', ( #6196, #779, #3380, #3858 ) ) ;
#4167=ORIENTED_EDGE ( 'NONE', *, *, #2225, .T. ) ;
#4168=LINE ( 'NONE', #6431, #1475 ) ;
#4169=ORIENTED_EDGE ( 'NONE', *, *, #2101, .F. ) ;
#4170=ADVANCED_FACE ( 'NONE', ( #3254 ), #5006, .F. ) ;
#4176=DIRECTION ( 'NONE',  ( 1.000000000000000000, 0.000000000000000000, 0.000000000000000000 ) ) ;
#4178=VERTEX_POINT ( 'NONE', #4808 ) ;
#4179=AXIS2_PLACEMENT_3D ( 'NONE', #4462, #1686, #1654 ) ;
#4188=ORIENTED_EDGE ( 'NONE', *, *, #193, .F. ) ;
#4196=CARTESIAN_POINT ( 'NONE',  ( 114.9999999999999858, -8.660254037844389075, 139.9990000000000236 ) ) ;
#4197=CARTESIAN_POINT ( 'NONE',  ( -30.00000000000002842, -20.00000000000000000, 140.0000000000000000 ) ) ;
#4199=EDGE_CURVE ( 'NONE', #2725, #1422, #1039, .T. ) ;
#4206=FACE_BOUND ( 'NONE', #6336, .T. ) ;
#4209=EDGE_CURVE ( 'NONE', #1367, #3461, #5980, .T. ) ;
#4213=LINE ( 'NONE', #4373, #1497 ) ;
#4224=ORIENTED_EDGE ( 'NONE', *, *, #1925, .F. ) ;
#4228=VERTEX_POINT ( 'NONE', #6171 ) ;
#4230=CARTESIAN_POINT ( 'NONE',  ( 435.0000000000000568, -8.660254037844389075, 145.0000000000000284 ) ) ;
#4234=LINE ( 'NONE', #4794, #3878 ) ;
#4236=CARTESIAN_POINT ( 'NONE',  ( 219.9999999999999716, -15.00000000000000000, 162.5000000000000853 ) ) ;
#4239=ORIENTED_EDGE ( 'NONE', *, *, #5485, .F. ) ;
#4241=EDGE_LOOP ( 'NONE', ( #1001, #4136, #3237, #2405 ) ) ;
#4244=AXIS2_PLACEMENT_3D ( 'NONE', #6104, #6509, #3647 ) ;
#4245=SURFACE_SIDE_STYLE ('',( #5976 ) ) ;
#4246=VECTOR ( 'NONE', #1522, 1000.000000000000000 ) ;
#4251=ORIENTED_EDGE ( 'NONE', *, *, #5997, .T. ) ;
#4253=DIRECTION ( 'NONE',  ( 0.000000000000000000, 1.000000000000000000, 0.000000000000000000 ) ) ;
#4254=CARTESIAN_POINT ( 'NONE',  ( 0.000000000000000000, 15.00000000000000000, 140.0000000000000000 ) ) ;
#4255=EDGE_CURVE ( 'NONE', #3309, #6561, #514, .T. ) ;
#4257=DIRECTION ( 'NONE',  ( 1.000000000000000000, 0.000000000000000000, 0.000000000000000000 ) ) ;
#4260=EDGE_CURVE ( 'NONE', #1596, #6322, #5505, .T. ) ;
#4261=DIRECTION ( 'NONE',  ( -0.000000000000000000, -0.000000000000000000, 1.000000000000000000 ) ) ;
#4268=VERTEX_POINT ( 'NONE', #6347 ) ;
#4277=ORIENTED_EDGE ( 'NONE', *, *, #4340, .T. ) ;
#4285=FACE_BOUND ( 'NONE', #247, .T. ) ;
#4287=EDGE_CURVE ( 'NONE', #3428, #5461, #4051, .T. ) ;
#4288=ORIENTED_EDGE ( 'NONE', *, *, #648, .F. ) ;
#4290=DIRECTION ( 'NONE',  ( 1.000000000000000000, 0.000000000000000000, 0.000000000000000000 ) ) ;
#4292=ORIENTED_EDGE ( 'NONE', *, *, #2403, .F. ) ;
#4293=ADVANCED_FACE ( 'NONE', ( #4584 ), #1766, .F. ) ;
#4297=FACE_BOUND ( 'NONE', #1877, .T. ) ;
#4299=ORIENTED_EDGE ( 'NONE', *, *, #4756, .T. ) ;
#4300=CARTESIAN_POINT ( 'NONE',  ( 405.0000000000000000, -8.660254037844389075, 140.0000000000000000 ) ) ;
#4302=ORIENTED_EDGE ( 'NONE', *, *, #6923, .F. ) ;
#4305=EDGE_CURVE ( 'NONE', #1731, #5144, #4085, .T. ) ;
#4306=DIRECTION ( 'NONE',  ( -0.000000000000000000, 1.000000000000000000, -0.000000000000000000 ) ) ;
#4314=EDGE_LOOP ( 'NONE', ( #2882, #7064, #2424, #2228 ) ) ;
#4316=CARTESIAN_POINT ( 'NONE',  ( 124.9999999999999858, 8.660254037844390851, 145.0000000000000284 ) ) ;
#4319=DIRECTION ( 'NONE',  ( 0.000000000000000000, 0.000000000000000000, 1.000000000000000000 ) ) ;
#4320=PRESENTATION_STYLE_ASSIGNMENT (( #2066 ) ) ;
#4322=CARTESIAN_POINT ( 'NONE',  ( 405.0000000000000000, 8.660254037844390851, 139.9990000000000236 ) ) ;
#4326=CARTESIAN_POINT ( 'NONE',  ( 325.0000000000000000, -8.660254037844389075, 139.9990000000000236 ) ) ;
#4327=AXIS2_PLACEMENT_3D ( 'NONE', #1969, #6673, #376 ) ;
#4333=VECTOR ( 'NONE', #999, 1000.000000000000000 ) ;
#4334=DIRECTION ( 'NONE',  ( -0.000000000000000000, 0.000000000000000000, 1.000000000000000000 ) ) ;
#4335=DIRECTION ( 'NONE',  ( -0.000000000000000000, 0.000000000000000000, -1.000000000000000000 ) ) ;
#4337=ORIENTED_EDGE ( 'NONE', *, *, #2728, .F. ) ;
#4340=EDGE_CURVE ( 'NONE', #3869, #7144, #2323, .T. ) ;
#4343=EDGE_CURVE ( 'NONE', #6959, #828, #2861, .T. ) ;
#4346=ORIENTED_EDGE ( 'NONE', *, *, #3033, .T. ) ;
#4354=CARTESIAN_POINT ( 'NONE',  ( 470.0000000000000000, 0.000000000000000000, 145.0000000000000284 ) ) ;
#4357=ORIENTED_EDGE ( 'NONE', *, *, #7216, .F. ) ;
#4363=CARTESIAN_POINT ( 'NONE',  ( 315.0000000000000568, -8.660254037844389075, 139.9990000000000236 ) ) ;
#4364=VECTOR ( 'NONE', #3943, 1000.000000000000000 ) ;
#4365=PLANE ( 'NONE',  #2778 ) ;
#4367=DIRECTION ( 'NONE',  ( -1.000000000000000000, -0.000000000000000000, -0.000000000000000000 ) ) ;
#4368=ORIENTED_EDGE ( 'NONE', *, *, #5799, .F. ) ;
#4372=AXIS2_PLACEMENT_3D ( 'NONE', #3516, #4624, #3446 ) ;
#4373=CARTESIAN_POINT ( 'NONE',  ( -5.000000000000000888, 8.660254037844390851, 140.0000000000000000 ) ) ;
#4374=ADVANCED_FACE ( 'NONE', ( #5118 ), #4519, .F. ) ;
#4377=AXIS2_PLACEMENT_3D ( 'NONE', #4644, #1758, #1786 ) ;
#4380=LINE ( 'NONE', #3192, #6484 ) ;
#4381=CARTESIAN_POINT ( 'NONE',  ( 35.00000000000000000, 8.660254037844390851, 140.0000000000000000 ) ) ;
#4387=VERTEX_POINT ( 'NONE', #1213 ) ;
#4388=AXIS2_PLACEMENT_3D ( 'NONE', #4805, #3796, #839 ) ;
#4389=EDGE_CURVE ( 'NONE', #1598, #1884, #2285, .T. ) ;
#4392=CARTESIAN_POINT ( 'NONE',  ( 235.0000000000000000, 8.660254037844390851, 139.9990000000000236 ) ) ;
#4399=ORIENTED_EDGE ( 'NONE', *, *, #1919, .T. ) ;
#4418=DIRECTION ( 'NONE',  ( -0.000000000000000000, -0.000000000000000000, 1.000000000000000000 ) ) ;
#4421=ORIENTED_EDGE ( 'NONE', *, *, #419, .F. ) ;
#4430=FACE_OUTER_BOUND ( 'NONE', #4166, .T. ) ;
#4432=CIRCLE ( 'NONE', #3367, 2.649999999999985700 ) ;
#4434=CARTESIAN_POINT ( 'NONE',  ( 470.0000000000000000, 15.00000000000000000, 145.0000000000000284 ) ) ;
#4447=DIRECTION ( 'NONE',  ( -1.000000000000000000, 0.000000000000000000, -0.000000000000000000 ) ) ;
#4455=DIRECTION ( 'NONE',  ( 0.000000000000000000, -1.000000000000000000, 0.000000000000000000 ) ) ;
#4460=ORIENTED_EDGE ( 'NONE', *, *, #1373, .T. ) ;
#4461=VERTEX_POINT ( 'NONE', #953 ) ;
#4462=CARTESIAN_POINT ( 'NONE',  ( 395.0000000000000000, 8.660254037844390851, 139.9990000000000236 ) ) ;
#4463=CARTESIAN_POINT ( 'NONE',  ( 45.00000000000000000, 8.660254037844390851, 145.0000000000000284 ) ) ;
#4465=LINE ( 'NONE', #1820, #1251 ) ;
#4470=LINE ( 'NONE', #6769, #5872 ) ;
#4473=ADVANCED_FACE ( 'NONE', ( #7248 ), #5472, .F. ) ;
#4474=AXIS2_PLACEMENT_3D ( 'NONE', #1604, #3886, #6182 ) ;
#4478=VECTOR ( 'NONE', #4290, 1000.000000000000000 ) ;
#4479=CARTESIAN_POINT ( 'NONE',  ( 470.0000000000000000, 15.00000000000000000, 140.0000000000000000 ) ) ;
#4488=DIRECTION ( 'NONE',  ( -0.000000000000000000, -0.000000000000000000, 1.000000000000000000 ) ) ;
#4489=ADVANCED_FACE ( 'NONE', ( #443 ), #323, .F. ) ;
#4491=AXIS2_PLACEMENT_3D ( 'NONE', #2797, #1056, #4566 ) ;
#4496=EDGE_CURVE ( 'NONE', #4971, #3920, #1588, .T. ) ;
#4500=ORIENTED_EDGE ( 'NONE', *, *, #4854, .F. ) ;
#4501=CARTESIAN_POINT ( 'NONE',  ( 325.0000000000000000, 8.660254037844390851, 139.9990000000000236 ) ) ;
#4512=CYLINDRICAL_SURFACE ( 'NONE', #1481, 2.649999999999985700 ) ;
#4513=LINE ( 'NONE', #6765, #6985 ) ;
#4519=PLANE ( 'NONE',  #3836 ) ;
#4520=CARTESIAN_POINT ( 'NONE',  ( 0.000000000000000000, 0.000000000000000000, 145.0000000000000284 ) ) ;
#4526=EDGE_LOOP ( 'NONE', ( #4591, #550, #5369, #226 ) ) ;
#4527=CARTESIAN_POINT ( 'NONE',  ( 315.0000000000000568, -8.660254037844389075, 139.9990000000000236 ) ) ;
#4529=EDGE_CURVE ( 'NONE', #6988, #6671, #1516, .T. ) ;
#4536=LINE ( 'NONE', #6827, #4757 ) ;
#4538=ORIENTED_EDGE ( 'NONE', *, *, #2365, .F. ) ;
#4542=LINE ( 'NONE', #6760, #6891 ) ;
#4543=ORIENTED_EDGE ( 'NONE', *, *, #6956, .T. ) ;
#4546=ORIENTED_EDGE ( 'NONE', *, *, #3186, .T. ) ;
#4549=CARTESIAN_POINT ( 'NONE',  ( 275.0000000000000000, 8.660254037844390851, 139.9990000000000236 ) ) ;
#4557=VERTEX_POINT ( 'NONE', #7203 ) ;
#4562=ORIENTED_EDGE ( 'NONE', *, *, #648, .T. ) ;
#4563=VECTOR ( 'NONE', #5355, 1000.000000000000000 ) ;
#4566=DIRECTION ( 'NONE',  ( 0.000000000000000000, 0.000000000000000000, 1.000000000000000000 ) ) ;
#4570=ORIENTED_EDGE ( 'NONE', *, *, #6789, .T. ) ;
#4572=FACE_OUTER_BOUND ( 'NONE', #4133, .T. ) ;
#4574=CARTESIAN_POINT ( 'NONE',  ( -5.000000000000000888, 8.660254037844390851, 140.0000000000000000 ) ) ;
#4578=ORIENTED_EDGE ( 'NONE', *, *, #2586, .T. ) ;
#4581=ORIENTED_EDGE ( 'NONE', *, *, #4734, .T. ) ;
#4582=DIRECTION ( 'NONE',  ( 0.000000000000000000, 1.000000000000000000, 0.000000000000000000 ) ) ;
#4584=FACE_OUTER_BOUND ( 'NONE', #3272, .T. ) ;
#4585=CARTESIAN_POINT ( 'NONE',  ( 435.0000000000000568, 8.660254037844390851, 145.0000000000000284 ) ) ;
#4588=ORIENTED_EDGE ( 'NONE', *, *, #6376, .T. ) ;
#4589=AXIS2_PLACEMENT_3D ( 'NONE', #2431, #5970, #3588 ) ;
#4591=ORIENTED_EDGE ( 'NONE', *, *, #4496, .T. ) ;
#4596=AXIS2_PLACEMENT_3D ( 'NONE', #6224, #535, #5106 ) ;
#4599=VERTEX_POINT ( 'NONE', #4316 ) ;
#4602=EDGE_CURVE ( 'NONE', #1207, #3032, #2141, .T. ) ;
#4612=CARTESIAN_POINT ( 'NONE',  ( 219.9999999999999716, -15.00000000000000000, 162.5000000000000853 ) ) ;
#4617=ORIENTED_EDGE ( 'NONE', *, *, #4152, .F. ) ;
#4622=EDGE_CURVE ( 'NONE', #3461, #5483, #1985, .T. ) ;
#4624=DIRECTION ( 'NONE',  ( 0.000000000000000000, 1.000000000000000000, 0.000000000000000000 ) ) ;
#4626=AXIS2_PLACEMENT_3D ( 'NONE', #5127, #7300, #39 ) ;
#4627=CARTESIAN_POINT ( 'NONE',  ( 235.0000000000000000, 8.660254037844390851, 140.0000000000000000 ) ) ;
#4631=ORIENTED_EDGE ( 'NONE', *, *, #2721, .F. ) ;
#4632=CIRCLE ( 'NONE', #1396, 2.649999999999985700 ) ;
#4633=DIRECTION ( 'NONE',  ( 0.000000000000000000, -0.000000000000000000, -1.000000000000000000 ) ) ;
#4635=ADVANCED_FACE ( 'NONE', ( #2844, #6237, #3445, #3414, #479, #5743 ), #6914, .F. ) ;
#4636=DIRECTION ( 'NONE',  ( 0.000000000000000000, 0.000000000000000000, 1.000000000000000000 ) ) ;
#4637=LINE ( 'NONE', #2958, #3888 ) ;
#4641=DIRECTION ( 'NONE',  ( 0.000000000000000000, 1.000000000000000000, 0.000000000000000000 ) ) ;
#4644=CARTESIAN_POINT ( 'NONE',  ( -5.000000000000000888, 8.660254037844390851, 139.9990000000000236 ) ) ;
#4645=DIRECTION ( 'NONE',  ( 0.000000000000000000, -1.000000000000000000, 0.000000000000000000 ) ) ;
#4650=DIRECTION ( 'NONE',  ( -0.000000000000000000, 1.000000000000000000, -0.000000000000000000 ) ) ;
#4652=CARTESIAN_POINT ( 'NONE',  ( 219.9999999999999716, -14.99999999999999822, 162.5000000000000853 ) ) ;
#4653=FACE_BOUND ( 'NONE', #372, .T. ) ;
#4655=FACE_OUTER_BOUND ( 'NONE', #4526, .T. ) ;
#4657=VERTEX_POINT ( 'NONE', #2813 ) ;
#4661=ADVANCED_FACE ( 'NONE', ( #2875 ), #4049, .F. ) ;
#4669=ORIENTED_EDGE ( 'NONE', *, *, #4622, .T. ) ;
#4678=LINE ( 'NONE', #5957, #4117 ) ;
#4680=CARTESIAN_POINT ( 'NONE',  ( 245.0000000000000000, -8.660254037844389075, 145.0000000000000284 ) ) ;
#4686=CARTESIAN_POINT ( 'NONE',  ( 84.99999999999998579, 8.660254037844390851, 140.0000000000000000 ) ) ;
#4689=VECTOR ( 'NONE', #4261, 1000.000000000000000 ) ;
#4693=ORIENTED_EDGE ( 'NONE', *, *, #2955, .T. ) ;
#4694=EDGE_CURVE ( 'NONE', #84, #1308, #4470, .T. ) ;
#4700=VECTOR ( 'NONE', #6548, 1000.000000000000000 ) ;
#4701=ORIENTED_EDGE ( 'NONE', *, *, #5619, .F. ) ;
#4702=ADVANCED_FACE ( 'NONE', ( #553 ), #6806, .F. ) ;
#4704=VECTOR ( 'NONE', #1676, 1000.000000000000000 ) ;
#4720=EDGE_LOOP ( 'NONE', ( #2122, #5749, #1114, #4807 ) ) ;
#4724=VECTOR ( 'NONE', #5523, 1000.000000000000000 ) ;
#4725=ORIENTED_EDGE ( 'NONE', *, *, #7080, .T. ) ;
#4726=ADVANCED_FACE ( 'NONE', ( #5817 ), #5215, .F. ) ;
#4730=LINE ( 'NONE', #4128, #3250 ) ;
#4734=EDGE_CURVE ( 'NONE', #2249, #7192, #1792, .T. ) ;
#4736=EDGE_LOOP ( 'NONE', ( #1586, #6943, #4368, #1642 ) ) ;
#4743=UNCERTAINTY_MEASURE_WITH_UNIT (LENGTH_MEASURE( 1.000000000000000082E-05 ), #2506, 'distance_accuracy_value', 'NONE');
#4746=PLANE ( 'NONE',  #1375 ) ;
#4750=ORIENTED_EDGE ( 'NONE', *, *, #6168, .T. ) ;
#4751=DIRECTION ( 'NONE',  ( 1.000000000000000000, 0.000000000000000000, 0.000000000000000000 ) ) ;
#4756=EDGE_CURVE ( 'NONE', #5845, #5499, #1346, .T. ) ;
#4757=VECTOR ( 'NONE', #1682, 1000.000000000000000 ) ;
#4758=VERTEX_POINT ( 'NONE', #1831 ) ;
#4760=DIRECTION ( 'NONE',  ( 0.000000000000000000, 0.000000000000000000, -1.000000000000000000 ) ) ;
#4761=DIRECTION ( 'NONE',  ( 0.000000000000000000, -1.000000000000000000, 0.000000000000000000 ) ) ;
#4764=FACE_OUTER_BOUND ( 'NONE', #6449, .T. ) ;
#4768=VERTEX_POINT ( 'NONE', #4083 ) ;
#4777=DIRECTION ( 'NONE',  ( -0.000000000000000000, -0.000000000000000000, 1.000000000000000000 ) ) ;
#4779=LINE ( 'NONE', #6511, #5822 ) ;
#4780=ORIENTED_EDGE ( 'NONE', *, *, #4255, .T. ) ;
#4781=ADVANCED_FACE ( 'NONE', ( #6973 ), #1934, .F. ) ;
#4782=LINE ( 'NONE', #261, #2045 ) ;
#4787=DIRECTION ( 'NONE',  ( -1.000000000000000000, 0.000000000000000000, 0.000000000000000000 ) ) ;
#4788=EDGE_LOOP ( 'NONE', ( #5508, #1229, #7055, #357 ) ) ;
#4791=CARTESIAN_POINT ( 'NONE',  ( 155.0000000000000000, -8.660254037844389075, 139.9990000000000236 ) ) ;
#4794=CARTESIAN_POINT ( 'NONE',  ( 315.0000000000000568, 8.660254037844390851, 139.9990000000000236 ) ) ;
#4798=EDGE_LOOP ( 'NONE', ( #3487, #6711, #4701, #5566 ) ) ;
#4805=CARTESIAN_POINT ( 'NONE',  ( 155.0000000000000000, 8.660254037844390851, 139.9990000000000236 ) ) ;
#4806=EDGE_LOOP ( 'NONE', ( #729, #5163, #6775, #3947 ) ) ;
#4807=ORIENTED_EDGE ( 'NONE', *, *, #5953, .F. ) ;
#4808=CARTESIAN_POINT ( 'NONE',  ( 4.999999999999999112, -8.660254037844389075, 145.0000000000000284 ) ) ;
#4812=VECTOR ( 'NONE', #6999, 1000.000000000000000 ) ;
#4814=CARTESIAN_POINT ( 'NONE',  ( 315.0000000000000568, 8.660254037844390851, 140.0000000000000000 ) ) ;
#4820=CARTESIAN_POINT ( 'NONE',  ( 303.3333333333333144, -15.00000000000000000, 165.1500000000000625 ) ) ;
#4821=PLANE ( 'NONE',  #1490 ) ;
#4823=AXIS2_PLACEMENT_3D ( 'NONE', #6842, #5082, #6282 ) ;
#4828=LINE ( 'NONE', #7120, #1437 ) ;
#4831=CARTESIAN_POINT ( 'NONE',  ( 195.0000000000000000, 8.660254037844390851, 145.0000000000000284 ) ) ;
#4833=FACE_OUTER_BOUND ( 'NONE', #245, .T. ) ;
#4834=EDGE_CURVE ( 'NONE', #3461, #6988, #206, .T. ) ;
#4837=EDGE_CURVE ( 'NONE', #584, #3428, #3626, .T. ) ;
#4840=LINE ( 'NONE', #7165, #776 ) ;
#4843=( LENGTH_UNIT ( ) NAMED_UNIT ( * ) SI_UNIT ( .MILLI., .METRE. ) );
#4850=CARTESIAN_POINT ( 'NONE',  ( 155.0000000000000000, 8.660254037844390851, 145.0000000000000284 ) ) ;
#4854=EDGE_CURVE ( 'NONE', #5461, #3920, #4159, .T. ) ;
#4859=FACE_OUTER_BOUND ( 'NONE', #5061, .T. ) ;
#4862=VERTEX_POINT ( 'NONE', #6450 ) ;
#4868=DIRECTION ( 'NONE',  ( -1.000000000000000000, 0.000000000000000000, -0.000000000000000000 ) ) ;
#4869=DIRECTION ( 'NONE',  ( -0.000000000000000000, -0.000000000000000000, 1.000000000000000000 ) ) ;
#4871=DIRECTION ( 'NONE',  ( -0.000000000000000000, 1.000000000000000000, 0.000000000000000000 ) ) ;
#4877=AXIS2_PLACEMENT_3D ( 'NONE', #1175, #3407, #583 ) ;
#4878=LINE ( 'NONE', #3754, #651 ) ;
#4879=ORIENTED_EDGE ( 'NONE', *, *, #3418, .T. ) ;
#4883=LINE ( 'NONE', #4322, #7121 ) ;
#4889=ADVANCED_FACE ( 'NONE', ( #2912 ), #2353, .F. ) ;
#4891=CARTESIAN_POINT ( 'NONE',  ( 53.33333333333330017, -15.00000000000000000, 162.5000000000000853 ) ) ;
#4892=ORIENTED_EDGE ( 'NONE', *, *, #1049, .F. ) ;
#4895=LINE ( 'NONE', #4820, #5765 ) ;
#4896=CARTESIAN_POINT ( 'NONE',  ( 124.9999999999999858, 8.660254037844390851, 139.9990000000000236 ) ) ;
#4908=LINE ( 'NONE', #863, #742 ) ;
#4912=DIRECTION ( 'NONE',  ( 0.000000000000000000, -0.000000000000000000, 1.000000000000000000 ) ) ;
#4914=ORIENTED_EDGE ( 'NONE', *, *, #4622, .F. ) ;
#4915=VECTOR ( 'NONE', #5778, 1000.000000000000000 ) ;
#4922=CARTESIAN_POINT ( 'NONE',  ( 365.0000000000000000, -8.660254037844389075, 140.0000000000000000 ) ) ;
#4927=ORIENTED_EDGE ( 'NONE', *, *, #694, .T. ) ;
#4930=DIRECTION ( 'NONE',  ( 0.000000000000000000, 1.000000000000000000, 0.000000000000000000 ) ) ;
#4931=CARTESIAN_POINT ( 'NONE',  ( 245.0000000000000000, -8.660254037844389075, 139.9990000000000236 ) ) ;
#4935=EDGE_CURVE ( 'NONE', #6744, #1168, #1505, .T. ) ;
#4937=VECTOR ( 'NONE', #6557, 1000.000000000000000 ) ;
#4939=DIRECTION ( 'NONE',  ( -0.000000000000000000, 0.000000000000000000, 1.000000000000000000 ) ) ;
#4941=ORIENTED_EDGE ( 'NONE', *, *, #1306, .T. ) ;
#4946=EDGE_CURVE ( 'NONE', #3722, #1084, #4828, .T. ) ;
#4949=ORIENTED_EDGE ( 'NONE', *, *, #7103, .F. ) ;
#4953=CARTESIAN_POINT ( 'NONE',  ( 405.0000000000000000, -8.660254037844389075, 139.9990000000000236 ) ) ;
#4957=DIRECTION ( 'NONE',  ( 0.000000000000000000, 0.000000000000000000, 1.000000000000000000 ) ) ;
#4959=ADVANCED_FACE ( 'NONE', ( #3663 ), #3737, .F. ) ;
#4965=CARTESIAN_POINT ( 'NONE',  ( 303.3333333333333144, -20.00000000000000000, 162.5000000000000853 ) ) ;
#4970=CARTESIAN_POINT ( 'NONE',  ( 235.0000000000000000, -8.660254037844389075, 139.9990000000000236 ) ) ;
#4971=VERTEX_POINT ( 'NONE', #6082 ) ;
#4975=VECTOR ( 'NONE', #2076, 1000.000000000000000 ) ;
#4979=CARTESIAN_POINT ( 'NONE',  ( 285.0000000000000568, -8.660254037844389075, 145.0000000000000284 ) ) ;
#4981=VECTOR ( 'NONE', #3976, 1000.000000000000000 ) ;
#4982=EDGE_LOOP ( 'NONE', ( #3765, #1052, #3442, #2449 ) ) ;
#4987=DIRECTION ( 'NONE',  ( 1.000000000000000000, 0.000000000000000000, 0.000000000000000000 ) ) ;
#4991=ORIENTED_EDGE ( 'NONE', *, *, #1115, .F. ) ;
#4994=VERTEX_POINT ( 'NONE', #7235 ) ;
#4995=DIRECTION ( 'NONE',  ( 1.000000000000000000, 0.000000000000000000, -0.000000000000000000 ) ) ;
#4999=LINE ( 'NONE', #6719, #6761 ) ;
#5003=VERTEX_POINT ( 'NONE', #6716 ) ;
#5005=CARTESIAN_POINT ( 'NONE',  ( -30.00000000000000000, 0.000000000000000000, 140.0000000000000000 ) ) ;
#5006=PLANE ( 'NONE',  #3214 ) ;
#5009=EDGE_CURVE ( 'NONE', #6725, #1598, #7194, .T. ) ;
#5011=EDGE_LOOP ( 'NONE', ( #2672, #7246, #3542, #6859 ) ) ;
#5012=DIRECTION ( 'NONE',  ( -1.000000000000000000, -0.000000000000000000, -0.000000000000000000 ) ) ;
#5015=ORIENTED_EDGE ( 'NONE', *, *, #2735, .F. ) ;
#5019=VERTEX_POINT ( 'NONE', #905 ) ;
#5020=CARTESIAN_POINT ( 'NONE',  ( -5.000000000000000888, -8.660254037844389075, 139.9990000000000236 ) ) ;
#5025=ORIENTED_EDGE ( 'NONE', *, *, #4946, .F. ) ;
#5030=CARTESIAN_POINT ( 'NONE',  ( 355.0000000000000000, -8.660254037844389075, 140.0000000000000000 ) ) ;
#5036=CARTESIAN_POINT ( 'NONE',  ( 235.0000000000000000, 8.660254037844390851, 145.0000000000000284 ) ) ;
#5037=ORIENTED_EDGE ( 'NONE', *, *, #1222, .F. ) ;
#5043=LINE ( 'NONE', #2067, #4333 ) ;
#5046=ORIENTED_EDGE ( 'NONE', *, *, #4059, .F. ) ;
#5048=EDGE_CURVE ( 'NONE', #5003, #2185, #2049, .T. ) ;
#5051=CARTESIAN_POINT ( 'NONE',  ( 445.0000000000000000, 8.660254037844390851, 139.9990000000000236 ) ) ;
#5055=CARTESIAN_POINT ( 'NONE',  ( 45.00000000000000000, -8.660254037844389075, 140.0000000000000000 ) ) ;
#5061=EDGE_LOOP ( 'NONE', ( #1110, #4357, #5926, #1152 ) ) ;
#5062=DIRECTION ( 'NONE',  ( -1.000000000000000000, 0.000000000000000000, 0.000000000000000000 ) ) ;
#5063=EDGE_CURVE ( 'NONE', #4768, #6751, #5603, .T. ) ;
#5064=ORIENTED_EDGE ( 'NONE', *, *, #5776, .T. ) ;
#5066=EDGE_LOOP ( 'NONE', ( #102, #2607, #2183, #7296 ) ) ;
#5070=CARTESIAN_POINT ( 'NONE',  ( 219.9999999999999716, -14.99999999999999822, 159.8500000000001080 ) ) ;
#5071=VECTOR ( 'NONE', #1868, 1000.000000000000000 ) ;
#5075=ORIENTED_EDGE ( 'NONE', *, *, #2791, .T. ) ;
#5076=AXIS2_PLACEMENT_3D ( 'NONE', #2412, #1785, #4073 ) ;
#5078=LINE ( 'NONE', #5005, #7247 ) ;
#5081=CARTESIAN_POINT ( 'NONE',  ( 136.6666666666666288, -20.00000000000000000, 162.5000000000000853 ) ) ;
#5082=DIRECTION ( 'NONE',  ( -0.000000000000000000, 1.000000000000000000, -0.000000000000000000 ) ) ;
#5086=CARTESIAN_POINT ( 'NONE',  ( 164.9999999999999716, 8.660254037844390851, 139.9990000000000236 ) ) ;
#5089=VERTEX_POINT ( 'NONE', #1616 ) ;
#5095=FACE_OUTER_BOUND ( 'NONE', #6446, .T. ) ;
#5106=DIRECTION ( 'NONE',  ( 0.000000000000000000, 0.000000000000000000, 1.000000000000000000 ) ) ;
#5109=AXIS2_PLACEMENT_3D ( 'NONE', #1655, #6641, #6682 ) ;
#5111=CARTESIAN_POINT ( 'NONE',  ( 303.3333333333333144, -20.00000000000000000, 159.8500000000001080 ) ) ;
#5112=CARTESIAN_POINT ( 'NONE',  ( 435.0000000000000568, 8.660254037844390851, 140.0000000000000000 ) ) ;
#5114=ORIENTED_EDGE ( 'NONE', *, *, #419, .T. ) ;
#5116=CARTESIAN_POINT ( 'NONE',  ( 0.000000000000000000, -20.00000000000000000, 0.000000000000000000 ) ) ;
#5118=FACE_OUTER_BOUND ( 'NONE', #3714, .T. ) ;
#5119=FACE_BOUND ( 'NONE', #604, .T. ) ;
#5121=ORIENTED_EDGE ( 'NONE', *, *, #3843, .F. ) ;
#5122=ORIENTED_EDGE ( 'NONE', *, *, #3248, .T. ) ;
#5125=EDGE_LOOP ( 'NONE', ( #1457, #1307, #3971, #5692 ) ) ;
#5126=CARTESIAN_POINT ( 'NONE',  ( 114.9999999999999858, 8.660254037844390851, 140.0000000000000000 ) ) ;
#5127=CARTESIAN_POINT ( 'NONE',  ( 45.00000000000000000, 8.660254037844390851, 139.9990000000000236 ) ) ;
#5130=ADVANCED_FACE ( 'NONE', ( #3286 ), #6158, .F. ) ;
#5135=ORIENTED_EDGE ( 'NONE', *, *, #4209, .T. ) ;
#5144=VERTEX_POINT ( 'NONE', #3403 ) ;
#5147=CARTESIAN_POINT ( 'NONE',  ( -5.000000000000000888, 8.660254037844390851, 139.9990000000000236 ) ) ;
#5149=DIRECTION ( 'NONE',  ( -0.000000000000000000, -0.000000000000000000, 1.000000000000000000 ) ) ;
#5152=ORIENTED_EDGE ( 'NONE', *, *, #2368, .T. ) ;
#5156=VECTOR ( 'NONE', #3870, 1000.000000000000000 ) ;
#5163=ORIENTED_EDGE ( 'NONE', *, *, #635, .T. ) ;
#5165=EDGE_CURVE ( 'NONE', #6755, #6469, #542, .T. ) ;
#5167=EDGE_LOOP ( 'NONE', ( #5522, #6792, #3160, #4927 ) ) ;
#5169=PLANE ( 'NONE',  #4377 ) ;
#5172=CARTESIAN_POINT ( 'NONE',  ( 155.0000000000000000, -8.660254037844389075, 145.0000000000000284 ) ) ;
#5173=VECTOR ( 'NONE', #3118, 1000.000000000000000 ) ;
#5174=ORIENTED_EDGE ( 'NONE', *, *, #6465, .F. ) ;
#5177=ORIENTED_EDGE ( 'NONE', *, *, #5695, .T. ) ;
#5179=FACE_OUTER_BOUND ( 'NONE', #5849, .T. ) ;
#5180=CARTESIAN_POINT ( 'NONE',  ( 45.00000000000000000, 8.660254037844390851, 145.0000000000000284 ) ) ;
#5186=ORIENTED_EDGE ( 'NONE', *, *, #4694, .T. ) ;
#5192=PLANE ( 'NONE',  #1975 ) ;
#5193=ORIENTED_EDGE ( 'NONE', *, *, #3536, .F. ) ;
#5194=AXIS2_PLACEMENT_3D ( 'NONE', #3440, #2808, #5738 ) ;
#5196=LINE ( 'NONE', #4143, #3764 ) ;
#5204=DIRECTION ( 'NONE',  ( 1.000000000000000000, 0.000000000000000000, 0.000000000000000000 ) ) ;
#5206=LINE ( 'NONE', #505, #2637 ) ;
#5212=ORIENTED_EDGE ( 'NONE', *, *, #6465, .T. ) ;
#5215=PLANE ( 'NONE',  #733 ) ;
#5216=LINE ( 'NONE', #99, #2688 ) ;
#5220=VECTOR ( 'NONE', #3268, 1000.000000000000000 ) ;
#5223=ORIENTED_EDGE ( 'NONE', *, *, #2179, .F. ) ;
#5224=ORIENTED_EDGE ( 'NONE', *, *, #4694, .F. ) ;
#5225=PRODUCT_CONTEXT ( 'NONE', #5493, 'mechanical' ) ;
#5226=DIRECTION ( 'NONE',  ( 0.000000000000000000, 1.000000000000000000, 0.000000000000000000 ) ) ;
#5234=DIRECTION ( 'NONE',  ( 0.000000000000000000, -0.000000000000000000, 1.000000000000000000 ) ) ;
#5237=LINE ( 'NONE', #5840, #2490 ) ;
#5239=FACE_OUTER_BOUND ( 'NONE', #2118, .T. ) ;
#5241=ORIENTED_EDGE ( 'NONE', *, *, #2815, .T. ) ;
#5245=DIRECTION ( 'NONE',  ( 0.000000000000000000, -0.000000000000000000, 1.000000000000000000 ) ) ;
#5246=DIRECTION ( 'NONE',  ( -0.000000000000000000, 1.000000000000000000, -0.000000000000000000 ) ) ;
#5248=CARTESIAN_POINT ( 'NONE',  ( 275.0000000000000000, 8.660254037844390851, 145.0000000000000284 ) ) ;
#5251=EDGE_CURVE ( 'NONE', #7046, #6469, #743, .T. ) ;
#5256=ORIENTED_EDGE ( 'NONE', *, *, #6360, .F. ) ;
#5257=VECTOR ( 'NONE', #2964, 1000.000000000000000 ) ;
#5261=ADVANCED_FACE ( 'NONE', ( #2898 ), #1334, .F. ) ;
#5266=VECTOR ( 'NONE', #6169, 1000.000000000000000 ) ;
#5267=ORIENTED_EDGE ( 'NONE', *, *, #3589, .T. ) ;
#5268=PLANE ( 'NONE',  #6790 ) ;
#5272=FACE_OUTER_BOUND ( 'NONE', #4314, .T. ) ;
#5273=CARTESIAN_POINT ( 'NONE',  ( 4.999999999999999112, 8.660254037844390851, 140.0000000000000000 ) ) ;
#5279=LINE ( 'NONE', #7045, #1811 ) ;
#5282=CARTESIAN_POINT ( 'NONE',  ( 315.0000000000000568, 8.660254037844390851, 145.0000000000000284 ) ) ;
#5287=PLANE ( 'NONE',  #4589 ) ;
#5291=DIRECTION ( 'NONE',  ( -1.000000000000000000, -0.000000000000000000, -0.000000000000000000 ) ) ;
#5292=ORIENTED_EDGE ( 'NONE', *, *, #7038, .T. ) ;
#5293=EDGE_CURVE ( 'NONE', #6744, #1972, #5237, .T. ) ;
#5303=CARTESIAN_POINT ( 'NONE',  ( 136.6666666666666288, -20.00000000000000000, 159.8500000000001080 ) ) ;
#5306=EDGE_CURVE ( 'NONE', #1084, #6398, #4432, .T. ) ;
#5313=EDGE_CURVE ( 'NONE', #1111, #4048, #3468, .T. ) ;
#5318=EDGE_LOOP ( 'NONE', ( #1892, #1011, #4543, #5241 ) ) ;
#5321=ORIENTED_EDGE ( 'NONE', *, *, #5466, .F. ) ;
#5324=DIRECTION ( 'NONE',  ( -0.000000000000000000, 0.000000000000000000, 1.000000000000000000 ) ) ;
#5327=CARTESIAN_POINT ( 'NONE',  ( 35.00000000000000000, 8.660254037844390851, 140.0000000000000000 ) ) ;
#5330=ORIENTED_EDGE ( 'NONE', *, *, #652, .F. ) ;
#5341=ORIENTED_EDGE ( 'NONE', *, *, #474, .F. ) ;
#5343=ADVANCED_FACE ( 'NONE', ( #5272 ), #6932, .F. ) ;
#5352=ORIENTED_EDGE ( 'NONE', *, *, #5997, .F. ) ;
#5353=EDGE_LOOP ( 'NONE', ( #6795, #3313, #4046, #3879 ) ) ;
#5355=DIRECTION ( 'NONE',  ( 0.000000000000000000, -1.000000000000000000, 0.000000000000000000 ) ) ;
#5357=LINE ( 'NONE', #6160, #5889 ) ;
#5359=EDGE_CURVE ( 'NONE', #1168, #6755, #3655, .T. ) ;
#5360=LINE ( 'NONE', #4196, #2661 ) ;
#5365=ORIENTED_EDGE ( 'NONE', *, *, #4199, .F. ) ;
#5369=ORIENTED_EDGE ( 'NONE', *, *, #1230, .F. ) ;
#5372=LINE ( 'NONE', #257, #642 ) ;
#5379=FACE_BOUND ( 'NONE', #1378, .T. ) ;
#5380=EDGE_CURVE ( 'NONE', #1873, #4461, #2520, .T. ) ;
#5381=ORIENTED_EDGE ( 'NONE', *, *, #5306, .T. ) ;
#5388=DIRECTION ( 'NONE',  ( 0.000000000000000000, -0.000000000000000000, -1.000000000000000000 ) ) ;
#5390=LINE ( 'NONE', #6490, #6038 ) ;
#5394=ORIENTED_EDGE ( 'NONE', *, *, #3853, .F. ) ;
#5402=CARTESIAN_POINT ( 'NONE',  ( 445.0000000000000000, -8.660254037844389075, 145.0000000000000284 ) ) ;
#5408=AXIS2_PLACEMENT_3D ( 'NONE', #2726, #6152, #5582 ) ;
#5417=CARTESIAN_POINT ( 'NONE',  ( 355.0000000000000000, -8.660254037844389075, 140.0000000000000000 ) ) ;
#5420=VECTOR ( 'NONE', #3290, 1000.000000000000000 ) ;
#5421=LINE ( 'NONE', #2043, #4937 ) ;
#5422=( GEOMETRIC_REPRESENTATION_CONTEXT ( 3 ) GLOBAL_UNCERTAINTY_ASSIGNED_CONTEXT ( ( #4743 ) ) GLOBAL_UNIT_ASSIGNED_CONTEXT ( ( #2506, #6610, #3175 ) ) REPRESENTATION_CONTEXT ( 'NONE', 'WORKASPACE' ) );
#5430=CARTESIAN_POINT ( 'NONE',  ( 53.33333333333330017, -15.00000000000000000, 159.8500000000001080 ) ) ;
#5433=VECTOR ( 'NONE', #2300, 1000.000000000000000 ) ;
#5437=DIRECTION ( 'NONE',  ( -0.000000000000000000, 1.000000000000000000, -0.000000000000000000 ) ) ;
#5438=ORIENTED_EDGE ( 'NONE', *, *, #1293, .T. ) ;
#5442=CARTESIAN_POINT ( 'NONE',  ( 205.0000000000000284, -8.660254037844389075, 145.0000000000000284 ) ) ;
#5451=LINE ( 'NONE', #4814, #2227 ) ;
#5454=CARTESIAN_POINT ( 'NONE',  ( 470.0000000000000000, -15.00000000000000000, 180.0000000000000284 ) ) ;
#5455=FACE_OUTER_BOUND ( 'NONE', #6090, .T. ) ;
#5456=CARTESIAN_POINT ( 'NONE',  ( 0.000000000000000000, 0.000000000000000000, 140.0000000000000000 ) ) ;
#5458=ORIENTED_EDGE ( 'NONE', *, *, #2864, .T. ) ;
#5461=VERTEX_POINT ( 'NONE', #3153 ) ;
#5466=EDGE_CURVE ( 'NONE', #3158, #818, #4782, .T. ) ;
#5467=LINE ( 'NONE', #910, #6390 ) ;
#5472=CYLINDRICAL_SURFACE ( 'NONE', #4071, 2.649999999999985700 ) ;
#5474=ORIENTED_EDGE ( 'NONE', *, *, #1014, .T. ) ;
#5477=FILL_AREA_STYLE ('',( #3675 ) ) ;
#5478=DIRECTION ( 'NONE',  ( 0.000000000000000000, -0.000000000000000000, 1.000000000000000000 ) ) ;
#5481=ORIENTED_EDGE ( 'NONE', *, *, #4837, .F. ) ;
#5483=VERTEX_POINT ( 'NONE', #5694 ) ;
#5484=DIRECTION ( 'NONE',  ( 0.000000000000000000, 0.000000000000000000, 1.000000000000000000 ) ) ;
#5485=EDGE_CURVE ( 'NONE', #1538, #732, #3429, .T. ) ;
#5491=DIRECTION ( 'NONE',  ( -0.000000000000000000, 1.000000000000000000, -0.000000000000000000 ) ) ;
#5493=APPLICATION_CONTEXT ( 'automotive_design' ) ;
#5498=ORIENTED_EDGE ( 'NONE', *, *, #2365, .T. ) ;
#5499=VERTEX_POINT ( 'NONE', #6745 ) ;
#5505=CIRCLE ( 'NONE', #5987, 2.649999999999985700 ) ;
#5508=ORIENTED_EDGE ( 'NONE', *, *, #6139, .T. ) ;
#5511=DIRECTION ( 'NONE',  ( 0.000000000000000000, 0.000000000000000000, 1.000000000000000000 ) ) ;
#5516=LINE ( 'NONE', #7100, #1166 ) ;
#5517=VECTOR ( 'NONE', #7186, 1000.000000000000000 ) ;
#5518=EDGE_LOOP ( 'NONE', ( #914, #1292, #952, #2645 ) ) ;
#5522=ORIENTED_EDGE ( 'NONE', *, *, #6846, .T. ) ;
#5523=DIRECTION ( 'NONE',  ( -0.000000000000000000, 1.000000000000000000, -0.000000000000000000 ) ) ;
#5527=ORIENTED_EDGE ( 'NONE', *, *, #2199, .T. ) ;
#5533=PLANE ( 'NONE',  #6046 ) ;
#5535=ORIENTED_EDGE ( 'NONE', *, *, #6699, .T. ) ;
#5538=MECHANICAL_DESIGN_GEOMETRIC_PRESENTATION_REPRESENTATION('',(#3378),#169);
#5545=EDGE_CURVE ( 'NONE', #6988, #6714, #2796, .T. ) ;
#5547=DIRECTION ( 'NONE',  ( -0.000000000000000000, 0.000000000000000000, 1.000000000000000000 ) ) ;
#5549=DIRECTION ( 'NONE',  ( 0.000000000000000000, -1.000000000000000000, 0.000000000000000000 ) ) ;
#5550=LINE ( 'NONE', #3863, #2676 ) ;
#5562=FACE_OUTER_BOUND ( 'NONE', #1662, .T. ) ;
#5566=ORIENTED_EDGE ( 'NONE', *, *, #7141, .F. ) ;
#5574=DIRECTION ( 'NONE',  ( 0.000000000000000000, 0.000000000000000000, 1.000000000000000000 ) ) ;
#5575=AXIS2_PLACEMENT_3D ( 'NONE', #4612, #2866, #3469 ) ;
#5578=FACE_OUTER_BOUND ( 'NONE', #2948, .T. ) ;
#5581=EDGE_LOOP ( 'NONE', ( #3980, #5075, #92, #4031 ) ) ;
#5582=DIRECTION ( 'NONE',  ( 0.000000000000000000, 0.000000000000000000, -1.000000000000000000 ) ) ;
#5591=CARTESIAN_POINT ( 'NONE',  ( 205.0000000000000284, 8.660254037844390851, 145.0000000000000284 ) ) ;
#5592=DIRECTION ( 'NONE',  ( -1.000000000000000000, 0.000000000000000000, 0.000000000000000000 ) ) ;
#5595=CARTESIAN_POINT ( 'NONE',  ( 136.6666666666666288, -15.00000000000000000, 162.5000000000000853 ) ) ;
#5603=LINE ( 'NONE', #5621, #6578 ) ;
#5604=ORIENTED_EDGE ( 'NONE', *, *, #7031, .T. ) ;
#5608=DIRECTION ( 'NONE',  ( -0.000000000000000000, 0.000000000000000000, 1.000000000000000000 ) ) ;
#5610=PLANE ( 'NONE',  #4474 ) ;
#5612=ORIENTED_EDGE ( 'NONE', *, *, #6730, .F. ) ;
#5614=CARTESIAN_POINT ( 'NONE',  ( 75.00000000000001421, -8.660254037844389075, 145.0000000000000284 ) ) ;
#5619=EDGE_CURVE ( 'NONE', #3869, #1933, #2683, .T. ) ;
#5620=ORIENTED_EDGE ( 'NONE', *, *, #1159, .T. ) ;
#5621=CARTESIAN_POINT ( 'NONE',  ( 275.0000000000000000, -8.660254037844389075, 139.9990000000000236 ) ) ;
#5625=CARTESIAN_POINT ( 'NONE',  ( 275.0000000000000000, 8.660254037844390851, 145.0000000000000284 ) ) ;
#5628=AXIS2_PLACEMENT_3D ( 'NONE', #272, #4995, #1458 ) ;
#5630=DIRECTION ( 'NONE',  ( 0.000000000000000000, -0.000000000000000000, 1.000000000000000000 ) ) ;
#5632=CARTESIAN_POINT ( 'NONE',  ( 315.0000000000000568, 8.660254037844390851, 139.9990000000000236 ) ) ;
#5633=FACE_OUTER_BOUND ( 'NONE', #6269, .T. ) ;
#5637=LINE ( 'NONE', #5086, #4096 ) ;
#5641=ORIENTED_EDGE ( 'NONE', *, *, #4935, .F. ) ;
#5648=VECTOR ( 'NONE', #3829, 1000.000000000000000 ) ;
#5653=EDGE_LOOP ( 'NONE', ( #6688, #3181 ) ) ;
#5654=LINE ( 'NONE', #2801, #2669 ) ;
#5658=DIRECTION ( 'NONE',  ( -1.000000000000000000, 0.000000000000000000, -0.000000000000000000 ) ) ;
#5660=CARTESIAN_POINT ( 'NONE',  ( 325.0000000000000000, -8.660254037844389075, 140.0000000000000000 ) ) ;
#5662=VECTOR ( 'NONE', #5934, 1000.000000000000000 ) ;
#5667=VECTOR ( 'NONE', #1906, 1000.000000000000000 ) ;
#5675=FACE_OUTER_BOUND ( 'NONE', #715, .T. ) ;
#5677=( NAMED_UNIT ( * ) PLANE_ANGLE_UNIT ( ) SI_UNIT ( $, .RADIAN. ) );
#5681=ORIENTED_EDGE ( 'NONE', *, *, #6441, .T. ) ;
#5685=ORIENTED_EDGE ( 'NONE', *, *, #1527, .F. ) ;
#5692=ORIENTED_EDGE ( 'NONE', *, *, #3639, .T. ) ;
#5693=AXIS2_PLACEMENT_3D ( 'NONE', #6727, #6840, #1664 ) ;
#5694=CARTESIAN_POINT ( 'NONE',  ( 365.0000000000000000, 8.660254037844390851, 145.0000000000000284 ) ) ;
#5695=EDGE_CURVE ( 'NONE', #2157, #3722, #4632, .T. ) ;
#5698=AXIS2_PLACEMENT_3D ( 'NONE', #1543, #434, #3404 ) ;
#5699=ORIENTED_EDGE ( 'NONE', *, *, #5825, .F. ) ;
#5708=LINE ( 'NONE', #1205, #1368 ) ;
#5714=CARTESIAN_POINT ( 'NONE',  ( -5.000000000000000888, -8.660254037844389075, 139.9990000000000236 ) ) ;
#5717=FACE_BOUND ( 'NONE', #5879, .T. ) ;
#5718=( NAMED_UNIT ( * ) SI_UNIT ( $, .STERADIAN. ) SOLID_ANGLE_UNIT ( ) );
#5723=DIRECTION ( 'NONE',  ( 0.000000000000000000, 0.000000000000000000, 1.000000000000000000 ) ) ;
#5725=EDGE_LOOP ( 'NONE', ( #135, #6705, #664, #1061 ) ) ;
#5726=DIRECTION ( 'NONE',  ( 1.000000000000000000, 0.000000000000000000, 0.000000000000000000 ) ) ;
#5730=ADVANCED_FACE ( 'NONE', ( #5562 ), #6772, .F. ) ;
#5733=CARTESIAN_POINT ( 'NONE',  ( 395.0000000000000000, 8.660254037844390851, 140.0000000000000000 ) ) ;
#5738=DIRECTION ( 'NONE',  ( 0.000000000000000000, 0.000000000000000000, -1.000000000000000000 ) ) ;
#5740=ORIENTED_EDGE ( 'NONE', *, *, #7320, .F. ) ;
#5743=FACE_OUTER_BOUND ( 'NONE', #3625, .T. ) ;
#5749=ORIENTED_EDGE ( 'NONE', *, *, #3432, .F. ) ;
#5754=ADVANCED_BREP_SHAPE_REPRESENTATION ( '', ( #3189, #1963 ), #5422 ) ;
#5756=AXIS2_PLACEMENT_3D ( 'NONE', #6841, #1737, #3951 ) ;
#5759=ORIENTED_EDGE ( 'NONE', *, *, #1919, .F. ) ;
#5765=VECTOR ( 'NONE', #1572, 1000.000000000000000 ) ;
#5770=LINE ( 'NONE', #90, #3856 ) ;
#5776=EDGE_CURVE ( 'NONE', #4178, #7027, #6729, .T. ) ;
#5777=VERTEX_POINT ( 'NONE', #446 ) ;
#5778=DIRECTION ( 'NONE',  ( 0.000000000000000000, -1.000000000000000000, 0.000000000000000000 ) ) ;
#5783=DIRECTION ( 'NONE',  ( 0.000000000000000000, -1.000000000000000000, 0.000000000000000000 ) ) ;
#5786=EDGE_LOOP ( 'NONE', ( #6156, #5814, #3080, #1268 ) ) ;
#5794=CARTESIAN_POINT ( 'NONE',  ( 315.0000000000000568, 8.660254037844390851, 140.0000000000000000 ) ) ;
#5799=EDGE_CURVE ( 'NONE', #2185, #4994, #6094, .T. ) ;
#5802=VECTOR ( 'NONE', #3071, 1000.000000000000000 ) ;
#5803=FACE_OUTER_BOUND ( 'NONE', #2983, .T. ) ;
#5806=DIRECTION ( 'NONE',  ( -0.000000000000000000, 1.000000000000000000, -0.000000000000000000 ) ) ;
#5810=CYLINDRICAL_SURFACE ( 'NONE', #6995, 2.649999999999985700 ) ;
#5814=ORIENTED_EDGE ( 'NONE', *, *, #3432, .T. ) ;
#5817=FACE_OUTER_BOUND ( 'NONE', #4788, .T. ) ;
#5822=VECTOR ( 'NONE', #708, 1000.000000000000000 ) ;
#5823=DIRECTION ( 'NONE',  ( 0.000000000000000000, -1.000000000000000000, 0.000000000000000000 ) ) ;
#5825=EDGE_CURVE ( 'NONE', #3722, #2157, #1684, .T. ) ;
#5826=VERTEX_POINT ( 'NONE', #1554 ) ;
#5827=CARTESIAN_POINT ( 'NONE',  ( 235.0000000000000000, 8.660254037844390851, 145.0000000000000284 ) ) ;
#5829=DIRECTION ( 'NONE',  ( 1.000000000000000000, 0.000000000000000000, 0.000000000000000000 ) ) ;
#5840=CARTESIAN_POINT ( 'NONE',  ( 470.0000000000000000, -20.00000000000000000, 180.0000000000000284 ) ) ;
#5845=VERTEX_POINT ( 'NONE', #2707 ) ;
#5848=ORIENTED_EDGE ( 'NONE', *, *, #2791, .F. ) ;
#5849=EDGE_LOOP ( 'NONE', ( #696, #5114, #5174, #6776 ) ) ;
#5856=ORIENTED_EDGE ( 'NONE', *, *, #5825, .T. ) ;
#5857=EDGE_CURVE ( 'NONE', #3377, #5019, #2427, .T. ) ;
#5859=CARTESIAN_POINT ( 'NONE',  ( 405.0000000000000000, -8.660254037844389075, 145.0000000000000284 ) ) ;
#5861=DIRECTION ( 'NONE',  ( 1.000000000000000000, 0.000000000000000000, 0.000000000000000000 ) ) ;
#5864=VERTEX_POINT ( 'NONE', #1698 ) ;
#5866=DIRECTION ( 'NONE',  ( -0.000000000000000000, -0.000000000000000000, 1.000000000000000000 ) ) ;
#5867=VECTOR ( 'NONE', #6839, 1000.000000000000000 ) ;
#5868=AXIS2_PLACEMENT_3D ( 'NONE', #4965, #1474, #4319 ) ;
#5872=VECTOR ( 'NONE', #1072, 1000.000000000000000 ) ;
#5873=CARTESIAN_POINT ( 'NONE',  ( 235.0000000000000000, 8.660254037844390851, 139.9990000000000236 ) ) ;
#5875=CARTESIAN_POINT ( 'NONE',  ( 136.6666666666666288, -15.00000000000000000, 159.8500000000001080 ) ) ;
#5879=EDGE_LOOP ( 'NONE', ( #1483, #612, #6588, #4421 ) ) ;
#5880=DIRECTION ( 'NONE',  ( 0.000000000000000000, 0.000000000000000000, -1.000000000000000000 ) ) ;
#5882=ORIENTED_EDGE ( 'NONE', *, *, #809, .T. ) ;
#5887=CARTESIAN_POINT ( 'NONE',  ( 365.0000000000000000, -8.660254037844389075, 145.0000000000000284 ) ) ;
#5889=VECTOR ( 'NONE', #2051, 1000.000000000000000 ) ;
#5890=ADVANCED_FACE ( 'NONE', ( #5633 ), #1076, .F. ) ;
#5894=ORIENTED_EDGE ( 'NONE', *, *, #4209, .F. ) ;
#5897=PLANE ( 'NONE',  #1971 ) ;
#5908=ORIENTED_EDGE ( 'NONE', *, *, #556, .F. ) ;
#5909=ORIENTED_EDGE ( 'NONE', *, *, #3778, .F. ) ;
#5915=VECTOR ( 'NONE', #2611, 1000.000000000000000 ) ;
#5916=ORIENTED_EDGE ( 'NONE', *, *, #7136, .T. ) ;
#5918=ADVANCED_FACE ( 'NONE', ( #2777, #2356, #5675, #4653, #6348, #3916, #1666, #6941, #5717, #5119, #1214, #515, #2286 ), #109, .F. ) ;
#5919=CARTESIAN_POINT ( 'NONE',  ( 285.0000000000000568, 8.660254037844390851, 145.0000000000000284 ) ) ;
#5923=VECTOR ( 'NONE', #5226, 1000.000000000000000 ) ;
#5926=ORIENTED_EDGE ( 'NONE', *, *, #6493, .F. ) ;
#5927=CIRCLE ( 'NONE', #4491, 2.649999999999985700 ) ;
#5934=DIRECTION ( 'NONE',  ( -0.000000000000000000, -0.000000000000000000, 1.000000000000000000 ) ) ;
#5935=DIRECTION ( 'NONE',  ( 0.000000000000000000, 0.000000000000000000, 1.000000000000000000 ) ) ;
#5937=EDGE_LOOP ( 'NONE', ( #201, #1844, #4780, #4631, #6957, #5152 ) ) ;
#5939=ORIENTED_EDGE ( 'NONE', *, *, #7145, .T. ) ;
#5942=DIRECTION ( 'NONE',  ( -1.000000000000000000, 0.000000000000000000, 0.000000000000000000 ) ) ;
#5945=EDGE_CURVE ( 'NONE', #1422, #7293, #6320, .T. ) ;
#5948=LINE ( 'NONE', #1075, #5648 ) ;
#5951=FACE_OUTER_BOUND ( 'NONE', #2544, .T. ) ;
#5953=EDGE_CURVE ( 'NONE', #4011, #1413, #5390, .T. ) ;
#5957=CARTESIAN_POINT ( 'NONE',  ( 245.0000000000000000, 8.660254037844390851, 145.0000000000000284 ) ) ;
#5965=EDGE_CURVE ( 'NONE', #5144, #6751, #3587, .T. ) ;
#5966=CARTESIAN_POINT ( 'NONE',  ( 470.0000000000000000, -20.00000000000000000, 180.0000000000000284 ) ) ;
#5967=LINE ( 'NONE', #7157, #564 ) ;
#5968=CARTESIAN_POINT ( 'NONE',  ( 365.0000000000000000, 8.660254037844390851, 140.0000000000000000 ) ) ;
#5970=DIRECTION ( 'NONE',  ( -0.000000000000000000, 1.000000000000000000, 0.000000000000000000 ) ) ;
#5971=CARTESIAN_POINT ( 'NONE',  ( -5.000000000000000888, 8.660254037844390851, 145.0000000000000284 ) ) ;
#5976=SURFACE_STYLE_FILL_AREA ( #5477 ) ;
#5977=DIRECTION ( 'NONE',  ( 0.000000000000000000, 1.000000000000000000, 0.000000000000000000 ) ) ;
#5979=ORIENTED_EDGE ( 'NONE', *, *, #4260, .F. ) ;
#5980=LINE ( 'NONE', #3300, #3093 ) ;
#5981=CARTESIAN_POINT ( 'NONE',  ( 219.9999999999999716, -15.00000000000000000, 165.1500000000000625 ) ) ;
#5984=DIRECTION ( 'NONE',  ( 0.000000000000000000, -1.000000000000000000, 0.000000000000000000 ) ) ;
#5986=ORIENTED_EDGE ( 'NONE', *, *, #1240, .F. ) ;
#5987=AXIS2_PLACEMENT_3D ( 'NONE', #4652, #1794, #2846 ) ;
#5990=CARTESIAN_POINT ( 'NONE',  ( 124.9999999999999858, -8.660254037844389075, 145.0000000000000284 ) ) ;
#5991=FACE_BOUND ( 'NONE', #2843, .T. ) ;
#5996=AXIS2_PLACEMENT_3D ( 'NONE', #690, #2942, #5245 ) ;
#5997=EDGE_CURVE ( 'NONE', #4387, #5845, #4234, .T. ) ;
#5998=ORIENTED_EDGE ( 'NONE', *, *, #2991, .T. ) ;
#6002=CARTESIAN_POINT ( 'NONE',  ( 195.0000000000000000, -8.660254037844389075, 139.9990000000000236 ) ) ;
#6008=AXIS2_PLACEMENT_3D ( 'NONE', #4150, #713, #6444 ) ;
#6018=ORIENTED_EDGE ( 'NONE', *, *, #5945, .F. ) ;
#6020=ORIENTED_EDGE ( 'NONE', *, *, #6493, .T. ) ;
#6022=CARTESIAN_POINT ( 'NONE',  ( 405.0000000000000000, 8.660254037844390851, 140.0000000000000000 ) ) ;
#6023=VECTOR ( 'NONE', #4164, 1000.000000000000000 ) ;
#6028=ORIENTED_EDGE ( 'NONE', *, *, #1527, .T. ) ;
#6034=DIRECTION ( 'NONE',  ( -1.000000000000000000, 0.000000000000000000, -0.000000000000000000 ) ) ;
#6037=VERTEX_POINT ( 'NONE', #3056 ) ;
#6038=VECTOR ( 'NONE', #2496, 1000.000000000000000 ) ;
#6039=FACE_OUTER_BOUND ( 'NONE', #3411, .T. ) ;
#6045=DIRECTION ( 'NONE',  ( 0.000000000000000000, 1.000000000000000000, 0.000000000000000000 ) ) ;
#6046=AXIS2_PLACEMENT_3D ( 'NONE', #3773, #2087, #4939 ) ;
#6048=DIRECTION ( 'NONE',  ( 1.000000000000000000, 0.000000000000000000, 0.000000000000000000 ) ) ;
#6049=CARTESIAN_POINT ( 'NONE',  ( 75.00000000000001421, 8.660254037844390851, 140.0000000000000000 ) ) ;
#6053=DIRECTION ( 'NONE',  ( -1.000000000000000000, -0.000000000000000000, -0.000000000000000000 ) ) ;
#6056=CIRCLE ( 'NONE', #4372, 2.649999999999985700 ) ;
#6060=EDGE_CURVE ( 'NONE', #1207, #7046, #275, .T. ) ;
#6061=CARTESIAN_POINT ( 'NONE',  ( 114.9999999999999858, 8.660254037844390851, 145.0000000000000284 ) ) ;
#6064=VERTEX_POINT ( 'NONE', #1869 ) ;
#6069=CARTESIAN_POINT ( 'NONE',  ( 235.0000000000000000, -8.660254037844389075, 140.0000000000000000 ) ) ;
#6071=ORIENTED_EDGE ( 'NONE', *, *, #6851, .F. ) ;
#6081=ORIENTED_EDGE ( 'NONE', *, *, #2864, .F. ) ;
#6082=CARTESIAN_POINT ( 'NONE',  ( 75.00000000000001421, -8.660254037844389075, 140.0000000000000000 ) ) ;
#6083=LINE ( 'NONE', #5030, #4137 ) ;
#6085=PLANE ( 'NONE',  #1244 ) ;
#6090=EDGE_LOOP ( 'NONE', ( #1217, #6616, #5908, #4224 ) ) ;
#6093=CARTESIAN_POINT ( 'NONE',  ( 245.0000000000000000, 8.660254037844390851, 140.0000000000000000 ) ) ;
#6094=LINE ( 'NONE', #3135, #7315 ) ;
#6096=PLANE ( 'NONE',  #2654 ) ;
#6100=ORIENTED_EDGE ( 'NONE', *, *, #7320, .T. ) ;
#6104=CARTESIAN_POINT ( 'NONE',  ( 315.0000000000000568, 8.660254037844390851, 139.9990000000000236 ) ) ;
#6105=CARTESIAN_POINT ( 'NONE',  ( 136.6666666666666288, -14.99999999999999822, 162.5000000000000853 ) ) ;
#6117=ORIENTED_EDGE ( 'NONE', *, *, #5048, .T. ) ;
#6132=DIRECTION ( 'NONE',  ( -0.000000000000000000, -0.000000000000000000, 1.000000000000000000 ) ) ;
#6139=EDGE_CURVE ( 'NONE', #2951, #2185, #1582, .T. ) ;
#6140=VECTOR ( 'NONE', #6048, 1000.000000000000000 ) ;
#6152=DIRECTION ( 'NONE',  ( 1.000000000000000000, 0.000000000000000000, 0.000000000000000000 ) ) ;
#6156=ORIENTED_EDGE ( 'NONE', *, *, #1153, .T. ) ;
#6157=ORIENTED_EDGE ( 'NONE', *, *, #1661, .T. ) ;
#6158=PLANE ( 'NONE',  #4179 ) ;
#6160=CARTESIAN_POINT ( 'NONE',  ( 386.6666666666666288, -15.00000000000000000, 165.1500000000000625 ) ) ;
#6162=VECTOR ( 'NONE', #2430, 1000.000000000000000 ) ;
#6168=EDGE_CURVE ( 'NONE', #5089, #5019, #909, .T. ) ;
#6169=DIRECTION ( 'NONE',  ( -0.000000000000000000, -0.000000000000000000, 1.000000000000000000 ) ) ;
#6170=DIRECTION ( 'NONE',  ( 0.000000000000000000, -1.000000000000000000, 0.000000000000000000 ) ) ;
#6171=CARTESIAN_POINT ( 'NONE',  ( 35.00000000000000000, 8.660254037844390851, 145.0000000000000284 ) ) ;
#6172=DIRECTION ( 'NONE',  ( 0.000000000000000000, -0.000000000000000000, -1.000000000000000000 ) ) ;
#6174=VECTOR ( 'NONE', #2444, 1000.000000000000000 ) ;
#6175=ORIENTED_EDGE ( 'NONE', *, *, #6789, .F. ) ;
#6182=DIRECTION ( 'NONE',  ( 0.000000000000000000, -0.000000000000000000, 1.000000000000000000 ) ) ;
#6184=EDGE_CURVE ( 'NONE', #3509, #4048, #4999, .T. ) ;
#6186=APPLICATION_CONTEXT ( 'automotive_design' ) ;
#6194=EDGE_CURVE ( 'NONE', #3982, #5845, #5550, .T. ) ;
#6196=ORIENTED_EDGE ( 'NONE', *, *, #6883, .T. ) ;
#6201=DIRECTION ( 'NONE',  ( -1.000000000000000000, -0.000000000000000000, -0.000000000000000000 ) ) ;
#6204=CARTESIAN_POINT ( 'NONE',  ( 84.99999999999998579, 8.660254037844390851, 140.0000000000000000 ) ) ;
#6215=LINE ( 'NONE', #2397, #6409 ) ;
#6217=ORIENTED_EDGE ( 'NONE', *, *, #5359, .F. ) ;
#6218=FACE_OUTER_BOUND ( 'NONE', #6869, .T. ) ;
#6223=ORIENTED_EDGE ( 'NONE', *, *, #7103, .T. ) ;
#6224=CARTESIAN_POINT ( 'NONE',  ( 53.33333333333330017, -20.00000000000000000, 162.5000000000000853 ) ) ;
#6230=EDGE_CURVE ( 'NONE', #3397, #4557, #6645, .T. ) ;
#6232=LINE ( 'NONE', #5036, #2071 ) ;
#6237=FACE_BOUND ( 'NONE', #383, .T. ) ;
#6239=CARTESIAN_POINT ( 'NONE',  ( 75.00000000000001421, 8.660254037844390851, 145.0000000000000284 ) ) ;
#6240=DIRECTION ( 'NONE',  ( -1.000000000000000000, 0.000000000000000000, 0.000000000000000000 ) ) ;
#6245=ORIENTED_EDGE ( 'NONE', *, *, #1159, .F. ) ;
#6256=DIRECTION ( 'NONE',  ( 1.000000000000000000, 0.000000000000000000, 0.000000000000000000 ) ) ;
#6258=EDGE_LOOP ( 'NONE', ( #4581, #5681, #7131, #5330 ) ) ;
#6267=CARTESIAN_POINT ( 'NONE',  ( 124.9999999999999858, 8.660254037844390851, 140.0000000000000000 ) ) ;
#6269=EDGE_LOOP ( 'NONE', ( #111, #5292, #576, #5193 ) ) ;
#6271=CARTESIAN_POINT ( 'NONE',  ( 315.0000000000000568, -8.660254037844389075, 140.0000000000000000 ) ) ;
#6273=AXIS2_PLACEMENT_3D ( 'NONE', #3205, #4871, #4912 ) ;
#6274=ADVANCED_FACE ( 'NONE', ( #3701 ), #6085, .F. ) ;
#6282=DIRECTION ( 'NONE',  ( 0.000000000000000000, 0.000000000000000000, 1.000000000000000000 ) ) ;
#6284=CARTESIAN_POINT ( 'NONE',  ( 75.00000000000001421, -8.660254037844389075, 139.9990000000000236 ) ) ;
#6286=VECTOR ( 'NONE', #2574, 1000.000000000000000 ) ;
#6289=ADVANCED_FACE ( 'NONE', ( #4017 ), #6801, .F. ) ;
#6291=ORIENTED_EDGE ( 'NONE', *, *, #6360, .T. ) ;
#6294=DIRECTION ( 'NONE',  ( -0.000000000000000000, -0.000000000000000000, 1.000000000000000000 ) ) ;
#6298=ORIENTED_EDGE ( 'NONE', *, *, #4021, .T. ) ;
#6302=CARTESIAN_POINT ( 'NONE',  ( 84.99999999999998579, -8.660254037844389075, 140.0000000000000000 ) ) ;
#6308=EDGE_LOOP ( 'NONE', ( #3064, #5474 ) ) ;
#6310=CIRCLE ( 'NONE', #1636, 2.649999999999985700 ) ;
#6314=ORIENTED_EDGE ( 'NONE', *, *, #3589, .F. ) ;
#6317=DIRECTION ( 'NONE',  ( 0.000000000000000000, -1.000000000000000000, 0.000000000000000000 ) ) ;
#6320=LINE ( 'NONE', #4585, #6162 ) ;
#6322=VERTEX_POINT ( 'NONE', #5070 ) ;
#6327=EDGE_CURVE ( 'NONE', #3673, #5144, #6341, .T. ) ;
#6334=VERTEX_POINT ( 'NONE', #6267 ) ;
#6336=EDGE_LOOP ( 'NONE', ( #7275, #4188 ) ) ;
#6337=DIRECTION ( 'NONE',  ( 0.000000000000000000, 0.000000000000000000, 1.000000000000000000 ) ) ;
#6341=LINE ( 'NONE', #5625, #3138 ) ;
#6347=CARTESIAN_POINT ( 'NONE',  ( 114.9999999999999858, -8.660254037844389075, 140.0000000000000000 ) ) ;
#6348=FACE_BOUND ( 'NONE', #3345, .T. ) ;
#6349=DIRECTION ( 'NONE',  ( 0.000000000000000000, -0.000000000000000000, -1.000000000000000000 ) ) ;
#6359=ORIENTED_EDGE ( 'NONE', *, *, #809, .F. ) ;
#6360=EDGE_CURVE ( 'NONE', #3466, #5483, #702, .T. ) ;
#6370=LINE ( 'NONE', #6408, #3412 ) ;
#6372=LINE ( 'NONE', #197, #7237 ) ;
#6376=EDGE_CURVE ( 'NONE', #4994, #1523, #5708, .T. ) ;
#6377=CARTESIAN_POINT ( 'NONE',  ( 155.0000000000000000, 8.660254037844390851, 140.0000000000000000 ) ) ;
#6378=ORIENTED_EDGE ( 'NONE', *, *, #3401, .T. ) ;
#6379=CARTESIAN_POINT ( 'NONE',  ( 355.0000000000000000, 8.660254037844390851, 140.0000000000000000 ) ) ;
#6381=DIRECTION ( 'NONE',  ( 1.000000000000000000, 0.000000000000000000, 0.000000000000000000 ) ) ;
#6384=PLANE ( 'NONE',  #2781 ) ;
#6390=VECTOR ( 'NONE', #3245, 1000.000000000000000 ) ;
#6392=CARTESIAN_POINT ( 'NONE',  ( 45.00000000000000000, 8.660254037844390851, 140.0000000000000000 ) ) ;
#6398=VERTEX_POINT ( 'NONE', #2869 ) ;
#6399=AXIS2_PLACEMENT_3D ( 'NONE', #5456, #4335, #3108 ) ;
#6404=VERTEX_POINT ( 'NONE', #5172 ) ;
#6406=VERTEX_POINT ( 'NONE', #5112 ) ;
#6408=CARTESIAN_POINT ( 'NONE',  ( 245.0000000000000000, 8.660254037844390851, 139.9990000000000236 ) ) ;
#6409=VECTOR ( 'NONE', #5861, 1000.000000000000000 ) ;
#6420=ORIENTED_EDGE ( 'NONE', *, *, #6796, .F. ) ;
#6423=DIRECTION ( 'NONE',  ( 0.000000000000000000, 0.000000000000000000, 1.000000000000000000 ) ) ;
#6424=LINE ( 'NONE', #1391, #6500 ) ;
#6428=ADVANCED_FACE ( 'NONE', ( #646 ), #7314, .F. ) ;
#6431=CARTESIAN_POINT ( 'NONE',  ( 325.0000000000000000, 8.660254037844390851, 140.0000000000000000 ) ) ;
#6437=CARTESIAN_POINT ( 'NONE',  ( 195.0000000000000000, 8.660254037844390851, 140.0000000000000000 ) ) ;
#6441=EDGE_CURVE ( 'NONE', #7192, #6404, #4542, .T. ) ;
#6444=DIRECTION ( 'NONE',  ( -0.000000000000000000, 0.000000000000000000, 1.000000000000000000 ) ) ;
#6446=EDGE_LOOP ( 'NONE', ( #1691, #2997, #2148, #3679 ) ) ;
#6449=EDGE_LOOP ( 'NONE', ( #4460, #5604, #6639, #4169 ) ) ;
#6450=CARTESIAN_POINT ( 'NONE',  ( 325.0000000000000000, -8.660254037844389075, 145.0000000000000284 ) ) ;
#6452=CARTESIAN_POINT ( 'NONE',  ( 84.99999999999998579, 8.660254037844390851, 145.0000000000000284 ) ) ;
#6455=EDGE_CURVE ( 'NONE', #1325, #7192, #4465, .T. ) ;
#6456=CYLINDRICAL_SURFACE ( 'NONE', #6977, 2.649999999999985700 ) ;
#6461=DIRECTION ( 'NONE',  ( 1.000000000000000000, 0.000000000000000000, 0.000000000000000000 ) ) ;
#6465=EDGE_CURVE ( 'NONE', #1782, #183, #3506, .T. ) ;
#6469=VERTEX_POINT ( 'NONE', #3541 ) ;
#6470=EDGE_LOOP ( 'NONE', ( #6018, #5365, #928, #3770 ) ) ;
#6473=LINE ( 'NONE', #1330, #4478 ) ;
#6476=VERTEX_POINT ( 'NONE', #685 ) ;
#6478=ADVANCED_FACE ( 'NONE', ( #5239 ), #5810, .F. ) ;
#6484=VECTOR ( 'NONE', #4418, 1000.000000000000000 ) ;
#6488=DIRECTION ( 'NONE',  ( 1.000000000000000000, 0.000000000000000000, 0.000000000000000000 ) ) ;
#6490=CARTESIAN_POINT ( 'NONE',  ( 195.0000000000000000, -8.660254037844389075, 145.0000000000000284 ) ) ;
#6493=EDGE_CURVE ( 'NONE', #1972, #3032, #6372, .T. ) ;
#6500=VECTOR ( 'NONE', #2429, 1000.000000000000000 ) ;
#6502=FACE_BOUND ( 'NONE', #5653, .T. ) ;
#6509=DIRECTION ( 'NONE',  ( -0.000000000000000000, 1.000000000000000000, 0.000000000000000000 ) ) ;
#6511=CARTESIAN_POINT ( 'NONE',  ( 275.0000000000000000, 8.660254037844390851, 140.0000000000000000 ) ) ;
#6513=EDGE_CURVE ( 'NONE', #2826, #767, #4678, .T. ) ;
#6522=ORIENTED_EDGE ( 'NONE', *, *, #1872, .T. ) ;
#6531=DIRECTION ( 'NONE',  ( -1.000000000000000000, 0.000000000000000000, 0.000000000000000000 ) ) ;
#6532=DIRECTION ( 'NONE',  ( -0.000000000000000000, 1.000000000000000000, -0.000000000000000000 ) ) ;
#6539=VECTOR ( 'NONE', #5984, 1000.000000000000000 ) ;
#6540=SHAPE_REPRESENTATION_RELATIONSHIP ( 'NONE' , 'NONE' ,  #3270, #5754 ) ;
#6542=ORIENTED_EDGE ( 'NONE', *, *, #3949, .F. ) ;
#6543=EDGE_LOOP ( 'NONE', ( #6902, #4588, #7117, #330 ) ) ;
#6548=DIRECTION ( 'NONE',  ( -0.000000000000000000, -0.000000000000000000, 1.000000000000000000 ) ) ;
#6550=DIRECTION ( 'NONE',  ( 1.000000000000000000, 0.000000000000000000, 0.000000000000000000 ) ) ;
#6553=FACE_BOUND ( 'NONE', #1893, .T. ) ;
#6557=DIRECTION ( 'NONE',  ( 0.000000000000000000, 1.000000000000000000, 0.000000000000000000 ) ) ;
#6561=VERTEX_POINT ( 'NONE', #3005 ) ;
#6564=CARTESIAN_POINT ( 'NONE',  ( 386.6666666666666288, -14.99999999999999822, 159.8500000000001080 ) ) ;
#6572=ORIENTED_EDGE ( 'NONE', *, *, #556, .T. ) ;
#6573=FACE_BOUND ( 'NONE', #561, .T. ) ;
#6577=FACE_OUTER_BOUND ( 'NONE', #3685, .T. ) ;
#6578=VECTOR ( 'NONE', #15, 1000.000000000000000 ) ;
#6579=CARTESIAN_POINT ( 'NONE',  ( 136.6666666666666288, -14.99999999999999822, 165.1500000000000625 ) ) ;
#6580=CYLINDRICAL_SURFACE ( 'NONE', #2105, 2.649999999999985700 ) ;
#6585=CARTESIAN_POINT ( 'NONE',  ( 195.0000000000000000, -8.660254037844389075, 140.0000000000000000 ) ) ;
#6588=ORIENTED_EDGE ( 'NONE', *, *, #3894, .F. ) ;
#6593=PRODUCT_DEFINITION_CONTEXT ( 'detailed design', #6186, 'design' ) ;
#6595=CARTESIAN_POINT ( 'NONE',  ( 35.00000000000000000, -8.660254037844389075, 145.0000000000000284 ) ) ;
#6605=CARTESIAN_POINT ( 'NONE',  ( 75.00000000000001421, -8.660254037844389075, 139.9990000000000236 ) ) ;
#6606=CARTESIAN_POINT ( 'NONE',  ( 386.6666666666666288, -20.00000000000000000, 159.8500000000001080 ) ) ;
#6610=( NAMED_UNIT ( * ) PLANE_ANGLE_UNIT ( ) SI_UNIT ( $, .RADIAN. ) );
#6612=DIRECTION ( 'NONE',  ( -0.000000000000000000, 1.000000000000000000, 0.000000000000000000 ) ) ;
#6614=FACE_OUTER_BOUND ( 'NONE', #1669, .T. ) ;
#6616=ORIENTED_EDGE ( 'NONE', *, *, #728, .T. ) ;
#6624=DIRECTION ( 'NONE',  ( -0.000000000000000000, 1.000000000000000000, -0.000000000000000000 ) ) ;
#6625=CARTESIAN_POINT ( 'NONE',  ( 205.0000000000000284, 8.660254037844390851, 140.0000000000000000 ) ) ;
#6631=ADVANCED_FACE ( 'NONE', ( #3811 ), #4821, .F. ) ;
#6637=VECTOR ( 'NONE', #6053, 1000.000000000000000 ) ;
#6639=ORIENTED_EDGE ( 'NONE', *, *, #920, .F. ) ;
#6641=DIRECTION ( 'NONE',  ( -0.000000000000000000, 1.000000000000000000, -0.000000000000000000 ) ) ;
#6645=LINE ( 'NONE', #6049, #5420 ) ;
#6647=DIRECTION ( 'NONE',  ( -0.000000000000000000, -0.000000000000000000, 1.000000000000000000 ) ) ;
#6650=AXIS2_PLACEMENT_3D ( 'NONE', #1487, #1157, #5608 ) ;
#6652=CIRCLE ( 'NONE', #1965, 2.649999999999985700 ) ;
#6653=DIRECTION ( 'NONE',  ( 0.000000000000000000, -0.000000000000000000, 1.000000000000000000 ) ) ;
#6656=( NAMED_UNIT ( * ) PLANE_ANGLE_UNIT ( ) SI_UNIT ( $, .RADIAN. ) );
#6659=CARTESIAN_POINT ( 'NONE',  ( 114.9999999999999858, 8.660254037844390851, 139.9990000000000236 ) ) ;
#6660=CARTESIAN_POINT ( 'NONE',  ( 164.9999999999999716, 8.660254037844390851, 145.0000000000000284 ) ) ;
#6668=VECTOR ( 'NONE', #110, 1000.000000000000000 ) ;
#6670=DIRECTION ( 'NONE',  ( -0.000000000000000000, -0.000000000000000000, 1.000000000000000000 ) ) ;
#6671=VERTEX_POINT ( 'NONE', #2562 ) ;
#6673=DIRECTION ( 'NONE',  ( -0.000000000000000000, 0.000000000000000000, 1.000000000000000000 ) ) ;
#6681=DIRECTION ( 'NONE',  ( 1.000000000000000000, 0.000000000000000000, 0.000000000000000000 ) ) ;
#6682=DIRECTION ( 'NONE',  ( 0.000000000000000000, 0.000000000000000000, 1.000000000000000000 ) ) ;
#6686=CARTESIAN_POINT ( 'NONE',  ( 53.33333333333330017, -15.00000000000000000, 162.5000000000000853 ) ) ;
#6688=ORIENTED_EDGE ( 'NONE', *, *, #1661, .F. ) ;
#6699=EDGE_CURVE ( 'NONE', #4862, #3982, #897, .T. ) ;
#6705=ORIENTED_EDGE ( 'NONE', *, *, #717, .F. ) ;
#6711=ORIENTED_EDGE ( 'NONE', *, *, #6796, .T. ) ;
#6713=ADVANCED_FACE ( 'NONE', ( #6553, #974, #4859, #1417, #3690, #3078, #5379, #264, #1535, #3231, #4297, #377, #5991 ), #3156, .T. ) ;
#6714=VERTEX_POINT ( 'NONE', #5417 ) ;
#6715=ORIENTED_EDGE ( 'NONE', *, *, #2995, .T. ) ;
#6716=CARTESIAN_POINT ( 'NONE',  ( 395.0000000000000000, -8.660254037844389075, 145.0000000000000284 ) ) ;
#6718=LINE ( 'NONE', #2573, #5173 ) ;
#6719=CARTESIAN_POINT ( 'NONE',  ( 124.9999999999999858, -8.660254037844389075, 139.9990000000000236 ) ) ;
#6721=VECTOR ( 'NONE', #6381, 1000.000000000000000 ) ;
#6725=VERTEX_POINT ( 'NONE', #304 ) ;
#6726=DIRECTION ( 'NONE',  ( -0.000000000000000000, -0.000000000000000000, -1.000000000000000000 ) ) ;
#6727=CARTESIAN_POINT ( 'NONE',  ( 219.9999999999999716, -20.00000000000000000, 162.5000000000000853 ) ) ;
#6729=LINE ( 'NONE', #1630, #1212 ) ;
#6730=EDGE_CURVE ( 'NONE', #3050, #3261, #2640, .T. ) ;
#6732=ADVANCED_FACE ( 'NONE', ( #1496 ), #5533, .F. ) ;
#6741=EDGE_CURVE ( 'NONE', #3920, #584, #1713, .T. ) ;
#6744=VERTEX_POINT ( 'NONE', #6857 ) ;
#6745=CARTESIAN_POINT ( 'NONE',  ( 315.0000000000000568, -8.660254037844389075, 145.0000000000000284 ) ) ;
#6748=CARTESIAN_POINT ( 'NONE',  ( 205.0000000000000284, 8.660254037844390851, 145.0000000000000284 ) ) ;
#6751=VERTEX_POINT ( 'NONE', #3276 ) ;
#6752=CARTESIAN_POINT ( 'NONE',  ( 395.0000000000000000, 8.660254037844390851, 140.0000000000000000 ) ) ;
#6755=VERTEX_POINT ( 'NONE', #601 ) ;
#6760=CARTESIAN_POINT ( 'NONE',  ( 155.0000000000000000, 8.660254037844390851, 145.0000000000000284 ) ) ;
#6761=VECTOR ( 'NONE', #2136, 1000.000000000000000 ) ;
#6765=CARTESIAN_POINT ( 'NONE',  ( 114.9999999999999858, 8.660254037844390851, 140.0000000000000000 ) ) ;
#6769=CARTESIAN_POINT ( 'NONE',  ( 445.0000000000000000, -8.660254037844389075, 139.9990000000000236 ) ) ;
#6770=LINE ( 'NONE', #2176, #559 ) ;
#6772=PLANE ( 'NONE',  #254 ) ;
#6774=DIRECTION ( 'NONE',  ( -0.000000000000000000, 1.000000000000000000, 0.000000000000000000 ) ) ;
#6775=ORIENTED_EDGE ( 'NONE', *, *, #3341, .F. ) ;
#6776=ORIENTED_EDGE ( 'NONE', *, *, #3401, .F. ) ;
#6779=ORIENTED_EDGE ( 'NONE', *, *, #1153, .F. ) ;
#6780=AXIS2_PLACEMENT_3D ( 'NONE', #2876, #63, #1793 ) ;
#6781=LINE ( 'NONE', #4527, #1623 ) ;
#6789=EDGE_CURVE ( 'NONE', #6755, #1207, #1087, .T. ) ;
#6790=AXIS2_PLACEMENT_3D ( 'NONE', #7071, #152, #5234 ) ;
#6792=ORIENTED_EDGE ( 'NONE', *, *, #3141, .T. ) ;
#6793=CARTESIAN_POINT ( 'NONE',  ( 114.9999999999999858, 8.660254037844390851, 145.0000000000000284 ) ) ;
#6795=ORIENTED_EDGE ( 'NONE', *, *, #3843, .T. ) ;
#6796=EDGE_CURVE ( 'NONE', #310, #1933, #2265, .T. ) ;
#6801=PLANE ( 'NONE',  #4877 ) ;
#6806=PLANE ( 'NONE',  #2390 ) ;
#6807=CARTESIAN_POINT ( 'NONE',  ( 395.0000000000000000, 8.660254037844390851, 145.0000000000000284 ) ) ;
#6809=DIRECTION ( 'NONE',  ( -0.000000000000000000, 0.000000000000000000, -1.000000000000000000 ) ) ;
#6817=CARTESIAN_POINT ( 'NONE',  ( 435.0000000000000568, -8.660254037844389075, 140.0000000000000000 ) ) ;
#6818=EDGE_CURVE ( 'NONE', #1413, #266, #44, .T. ) ;
#6819=CARTESIAN_POINT ( 'NONE',  ( 219.9999999999999716, -14.99999999999999822, 162.5000000000000853 ) ) ;
#6827=CARTESIAN_POINT ( 'NONE',  ( 355.0000000000000000, -8.660254037844389075, 145.0000000000000284 ) ) ;
#6831=CARTESIAN_POINT ( 'NONE',  ( 470.0000000000000000, -20.00000000000000000, 140.0000000000000000 ) ) ;
#6838=ORIENTED_EDGE ( 'NONE', *, *, #1444, .T. ) ;
#6839=DIRECTION ( 'NONE',  ( -0.000000000000000000, -0.000000000000000000, 1.000000000000000000 ) ) ;
#6840=DIRECTION ( 'NONE',  ( 0.000000000000000000, 1.000000000000000000, 0.000000000000000000 ) ) ;
#6841=CARTESIAN_POINT ( 'NONE',  ( 303.3333333333333144, -15.00000000000000000, 162.5000000000000853 ) ) ;
#6842=CARTESIAN_POINT ( 'NONE',  ( 53.33333333333330017, -14.99999999999999822, 162.5000000000000853 ) ) ;
#6845=LINE ( 'NONE', #2916, #3865 ) ;
#6846=EDGE_CURVE ( 'NONE', #2062, #3817, #3430, .T. ) ;
#6851=EDGE_CURVE ( 'NONE', #4048, #4599, #3318, .T. ) ;
#6853=LINE ( 'NONE', #2825, #2445 ) ;
#6857=CARTESIAN_POINT ( 'NONE',  ( 470.0000000000000000, -20.00000000000000000, 180.0000000000000284 ) ) ;
#6859=ORIENTED_EDGE ( 'NONE', *, *, #5485, .T. ) ;
#6862=EDGE_CURVE ( 'NONE', #1770, #7340, #5927, .T. ) ;
#6863=ORIENTED_EDGE ( 'NONE', *, *, #948, .T. ) ;
#6865=CYLINDRICAL_SURFACE ( 'NONE', #5575, 2.649999999999985700 ) ;
#6869=EDGE_LOOP ( 'NONE', ( #5186, #3472, #4288, #3789 ) ) ;
#6875=VERTEX_POINT ( 'NONE', #6302 ) ;
#6879=DIRECTION ( 'NONE',  ( -0.000000000000000000, 1.000000000000000000, -0.000000000000000000 ) ) ;
#6881=VECTOR ( 'NONE', #7012, 1000.000000000000000 ) ;
#6883=EDGE_CURVE ( 'NONE', #3397, #3428, #6897, .T. ) ;
#6884=CARTESIAN_POINT ( 'NONE',  ( 155.0000000000000000, -8.660254037844389075, 140.0000000000000000 ) ) ;
#6891=VECTOR ( 'NONE', #2313, 1000.000000000000000 ) ;
#6893=CIRCLE ( 'NONE', #898, 2.649999999999985700 ) ;
#6897=LINE ( 'NONE', #1646, #3405 ) ;
#6902=ORIENTED_EDGE ( 'NONE', *, *, #1414, .T. ) ;
#6907=CARTESIAN_POINT ( 'NONE',  ( 395.0000000000000000, -8.660254037844389075, 140.0000000000000000 ) ) ;
#6910=ORIENTED_EDGE ( 'NONE', *, *, #2815, .F. ) ;
#6914=PLANE ( 'NONE',  #2625 ) ;
#6916=DIRECTION ( 'NONE',  ( 0.000000000000000000, 1.000000000000000000, 0.000000000000000000 ) ) ;
#6919=ORIENTED_EDGE ( 'NONE', *, *, #1613, .F. ) ;
#6923=EDGE_CURVE ( 'NONE', #5777, #3673, #4637, .T. ) ;
#6926=EDGE_CURVE ( 'NONE', #2205, #1598, #4064, .T. ) ;
#6927=DIRECTION ( 'NONE',  ( -0.000000000000000000, 1.000000000000000000, -0.000000000000000000 ) ) ;
#6931=ORIENTED_EDGE ( 'NONE', *, *, #2234, .F. ) ;
#6932=PLANE ( 'NONE',  #5076 ) ;
#6933=CARTESIAN_POINT ( 'NONE',  ( -30.00000000000002842, -20.00000000000000000, 140.0000000000000000 ) ) ;
#6937=EDGE_LOOP ( 'NONE', ( #5177, #5856 ) ) ;
#6938=CARTESIAN_POINT ( 'NONE',  ( 75.00000000000001421, 8.660254037844390851, 145.0000000000000284 ) ) ;
#6940=CARTESIAN_POINT ( 'NONE',  ( -5.000000000000000888, -8.660254037844389075, 140.0000000000000000 ) ) ;
#6941=FACE_BOUND ( 'NONE', #4081, .T. ) ;
#6943=ORIENTED_EDGE ( 'NONE', *, *, #6376, .F. ) ;
#6946=CARTESIAN_POINT ( 'NONE',  ( 219.9999999999999716, -20.00000000000000000, 159.8500000000001080 ) ) ;
#6955=LINE ( 'NONE', #2402, #2911 ) ;
#6956=EDGE_CURVE ( 'NONE', #818, #6064, #737, .T. ) ;
#6957=ORIENTED_EDGE ( 'NONE', *, *, #5251, .F. ) ;
#6959=VERTEX_POINT ( 'NONE', #5303 ) ;
#6960=AXIS2_PLACEMENT_3D ( 'NONE', #2039, #6034, #4334 ) ;
#6965=LINE ( 'NONE', #5875, #738 ) ;
#6966=CARTESIAN_POINT ( 'NONE',  ( 386.6666666666666288, -15.00000000000000000, 162.5000000000000853 ) ) ;
#6972=ORIENTED_EDGE ( 'NONE', *, *, #4602, .T. ) ;
#6973=FACE_OUTER_BOUND ( 'NONE', #307, .T. ) ;
#6977=AXIS2_PLACEMENT_3D ( 'NONE', #4236, #6532, #726 ) ;
#6981=VECTOR ( 'NONE', #1532, 1000.000000000000000 ) ;
#6985=VECTOR ( 'NONE', #2280, 1000.000000000000000 ) ;
#6988=VERTEX_POINT ( 'NONE', #777 ) ;
#6991=DIRECTION ( 'NONE',  ( -1.000000000000000000, 0.000000000000000000, 0.000000000000000000 ) ) ;
#6993=ORIENTED_EDGE ( 'NONE', *, *, #2003, .T. ) ;
#6995=AXIS2_PLACEMENT_3D ( 'NONE', #6966, #3657, #2936 ) ;
#6998=LINE ( 'NONE', #1851, #6174 ) ;
#6999=DIRECTION ( 'NONE',  ( 0.000000000000000000, 1.000000000000000000, 0.000000000000000000 ) ) ;
#7012=DIRECTION ( 'NONE',  ( 0.000000000000000000, -1.000000000000000000, 0.000000000000000000 ) ) ;
#7020=DIRECTION ( 'NONE',  ( -0.000000000000000000, -0.000000000000000000, 1.000000000000000000 ) ) ;
#7026=FACE_OUTER_BOUND ( 'NONE', #6258, .T. ) ;
#7027=VERTEX_POINT ( 'NONE', #7067 ) ;
#7030=EDGE_LOOP ( 'NONE', ( #5122, #161, #6779, #7065 ) ) ;
#7031=EDGE_CURVE ( 'NONE', #3206, #2826, #6955, .T. ) ;
#7038=EDGE_CURVE ( 'NONE', #2383, #1770, #5196, .T. ) ;
#7045=CARTESIAN_POINT ( 'NONE',  ( 136.6666666666666288, -15.00000000000000000, 165.1500000000000625 ) ) ;
#7046=VERTEX_POINT ( 'NONE', #1196 ) ;
#7055=ORIENTED_EDGE ( 'NONE', *, *, #1414, .F. ) ;
#7064=ORIENTED_EDGE ( 'NONE', *, *, #5313, .T. ) ;
#7065=ORIENTED_EDGE ( 'NONE', *, *, #2955, .F. ) ;
#7067=CARTESIAN_POINT ( 'NONE',  ( 4.999999999999999112, 8.660254037844390851, 145.0000000000000284 ) ) ;
#7068=AXIS2_PLACEMENT_3D ( 'NONE', #3207, #2704, #6653 ) ;
#7069=ORIENTED_EDGE ( 'NONE', *, *, #3778, .T. ) ;
#7071=CARTESIAN_POINT ( 'NONE',  ( 35.00000000000000000, 8.660254037844390851, 139.9990000000000236 ) ) ;
#7072=ORIENTED_EDGE ( 'NONE', *, *, #3853, .T. ) ;
#7080=EDGE_CURVE ( 'NONE', #6334, #4599, #6998, .T. ) ;
#7089=LINE ( 'NONE', #1942, #7101 ) ;
#7093=ADVANCED_FACE ( 'NONE', ( #1297 ), #4746, .F. ) ;
#7099=LINE ( 'NONE', #5827, #291 ) ;
#7100=CARTESIAN_POINT ( 'NONE',  ( 435.0000000000000568, -8.660254037844389075, 139.9990000000000236 ) ) ;
#7101=VECTOR ( 'NONE', #3668, 1000.000000000000000 ) ;
#7103=EDGE_CURVE ( 'NONE', #828, #6959, #6893, .T. ) ;
#7104=ORIENTED_EDGE ( 'NONE', *, *, #6956, .F. ) ;
#7112=CARTESIAN_POINT ( 'NONE',  ( 445.0000000000000000, 8.660254037844390851, 140.0000000000000000 ) ) ;
#7115=ORIENTED_EDGE ( 'NONE', *, *, #6851, .T. ) ;
#7117=ORIENTED_EDGE ( 'NONE', *, *, #3033, .F. ) ;
#7118=VECTOR ( 'NONE', #4488, 1000.000000000000000 ) ;
#7119=EDGE_LOOP ( 'NONE', ( #441, #2279, #2754, #4337 ) ) ;
#7120=CARTESIAN_POINT ( 'NONE',  ( 303.3333333333333144, -15.00000000000000000, 159.8500000000001080 ) ) ;
#7121=VECTOR ( 'NONE', #6132, 1000.000000000000000 ) ;
#7131=ORIENTED_EDGE ( 'NONE', *, *, #1710, .F. ) ;
#7134=( NAMED_UNIT ( * ) SI_UNIT ( $, .STERADIAN. ) SOLID_ANGLE_UNIT ( ) );
#7136=EDGE_CURVE ( 'NONE', #6037, #1596, #3220, .T. ) ;
#7138=ORIENTED_EDGE ( 'NONE', *, *, #1690, .T. ) ;
#7141=EDGE_CURVE ( 'NONE', #3826, #3869, #4213, .T. ) ;
#7142=FACE_OUTER_BOUND ( 'NONE', #1890, .T. ) ;
#7144=VERTEX_POINT ( 'NONE', #409 ) ;
#7145=EDGE_CURVE ( 'NONE', #3261, #1397, #3183, .T. ) ;
#7155=VERTEX_POINT ( 'NONE', #367 ) ;
#7157=CARTESIAN_POINT ( 'NONE',  ( 405.0000000000000000, 8.660254037844390851, 140.0000000000000000 ) ) ;
#7158=CARTESIAN_POINT ( 'NONE',  ( 285.0000000000000568, 8.660254037844390851, 145.0000000000000284 ) ) ;
#7165=CARTESIAN_POINT ( 'NONE',  ( 445.0000000000000000, 8.660254037844390851, 145.0000000000000284 ) ) ;
#7167=DIRECTION ( 'NONE',  ( 0.000000000000000000, -1.000000000000000000, 0.000000000000000000 ) ) ;
#7175=ORIENTED_EDGE ( 'NONE', *, *, #5857, .F. ) ;
#7178=CARTESIAN_POINT ( 'NONE',  ( 219.9999999999999716, -20.00000000000000000, 162.5000000000000853 ) ) ;
#7179=DIRECTION ( 'NONE',  ( 0.000000000000000000, -1.000000000000000000, 0.000000000000000000 ) ) ;
#7181=VECTOR ( 'NONE', #3681, 1000.000000000000000 ) ;
#7186=DIRECTION ( 'NONE',  ( 1.000000000000000000, 0.000000000000000000, 0.000000000000000000 ) ) ;
#7192=VERTEX_POINT ( 'NONE', #4850 ) ;
#7194=LINE ( 'NONE', #6595, #2621 ) ;
#7195=PLANE ( 'NONE',  #5698 ) ;
#7196=LINE ( 'NONE', #388, #6140 ) ;
#7198=LINE ( 'NONE', #3908, #58 ) ;
#7203=CARTESIAN_POINT ( 'NONE',  ( 75.00000000000001421, 8.660254037844390851, 140.0000000000000000 ) ) ;
#7205=ORIENTED_EDGE ( 'NONE', *, *, #4946, .T. ) ;
#7208=PLANE ( 'NONE',  #4388 ) ;
#7209=VECTOR ( 'NONE', #1593, 1000.000000000000000 ) ;
#7214=LINE ( 'NONE', #4254, #4975 ) ;
#7216=EDGE_CURVE ( 'NONE', #3032, #2165, #7214, .T. ) ;
#7223=VECTOR ( 'NONE', #3910, 1000.000000000000000 ) ;
#7228=ORIENTED_EDGE ( 'NONE', *, *, #3702, .T. ) ;
#7232=ADVANCED_FACE ( 'NONE', ( #6577 ), #1442, .F. ) ;
#7234=VERTEX_POINT ( 'NONE', #6069 ) ;
#7235=CARTESIAN_POINT ( 'NONE',  ( 405.0000000000000000, 8.660254037844390851, 145.0000000000000284 ) ) ;
#7237=VECTOR ( 'NONE', #4116, 1000.000000000000000 ) ;
#7244=EDGE_CURVE ( 'NONE', #3697, #4862, #814, .T. ) ;
#7246=ORIENTED_EDGE ( 'NONE', *, *, #2101, .T. ) ;
#7247=VECTOR ( 'NONE', #954, 1000.000000000000000 ) ;
#7248=FACE_OUTER_BOUND ( 'NONE', #2074, .T. ) ;
#7250=DIRECTION ( 'NONE',  ( 0.000000000000000000, 0.000000000000000000, 1.000000000000000000 ) ) ;
#7256=CARTESIAN_POINT ( 'NONE',  ( 355.0000000000000000, 8.660254037844390851, 145.0000000000000284 ) ) ;
#7258=VERTEX_POINT ( 'NONE', #6022 ) ;
#7263=ADVANCED_FACE ( 'NONE', ( #3100 ), #888, .F. ) ;
#7275=ORIENTED_EDGE ( 'NONE', *, *, #2840, .F. ) ;
#7280=EDGE_CURVE ( 'NONE', #1523, #5003, #596, .T. ) ;
#7290=EDGE_CURVE ( 'NONE', #6714, #7155, #3425, .T. ) ;
#7293=VERTEX_POINT ( 'NONE', #491 ) ;
#7296=ORIENTED_EDGE ( 'NONE', *, *, #3973, .F. ) ;
#7300=DIRECTION ( 'NONE',  ( 1.000000000000000000, 0.000000000000000000, 0.000000000000000000 ) ) ;
#7305=DIRECTION ( 'NONE',  ( -0.000000000000000000, 1.000000000000000000, -0.000000000000000000 ) ) ;
#7307=VERTEX_POINT ( 'NONE', #5126 ) ;
#7314=PLANE ( 'NONE',  #5194 ) ;
#7315=VECTOR ( 'NONE', #955, 1000.000000000000000 ) ;
#7320=EDGE_CURVE ( 'NONE', #2711, #5499, #6781, .T. ) ;
#7328=DIRECTION ( 'NONE',  ( 1.000000000000000000, 0.000000000000000000, 0.000000000000000000 ) ) ;
#7338=DIRECTION ( 'NONE',  ( 0.000000000000000000, 0.000000000000000000, 1.000000000000000000 ) ) ;
#7340=VERTEX_POINT ( 'NONE', #3266 ) ;
#7419=COLOUR_RGB('Light Blue',0.38,0.62,0.78);
#7420=FILL_AREA_STYLE_COLOUR('',#7419);
#7421=FILL_AREA_STYLE('',(#7420));
#7422=SURFACE_STYLE_FILL_AREA(#7421);
#7423=SURFACE_SIDE_STYLE('',(#7422));
#7424=SURFACE_STYLE_USAGE(.BOTH.,#7423);
#7425=PRESENTATION_STYLE_ASSIGNMENT((#7424));
ENDSEC;
END-ISO-10303-21;
